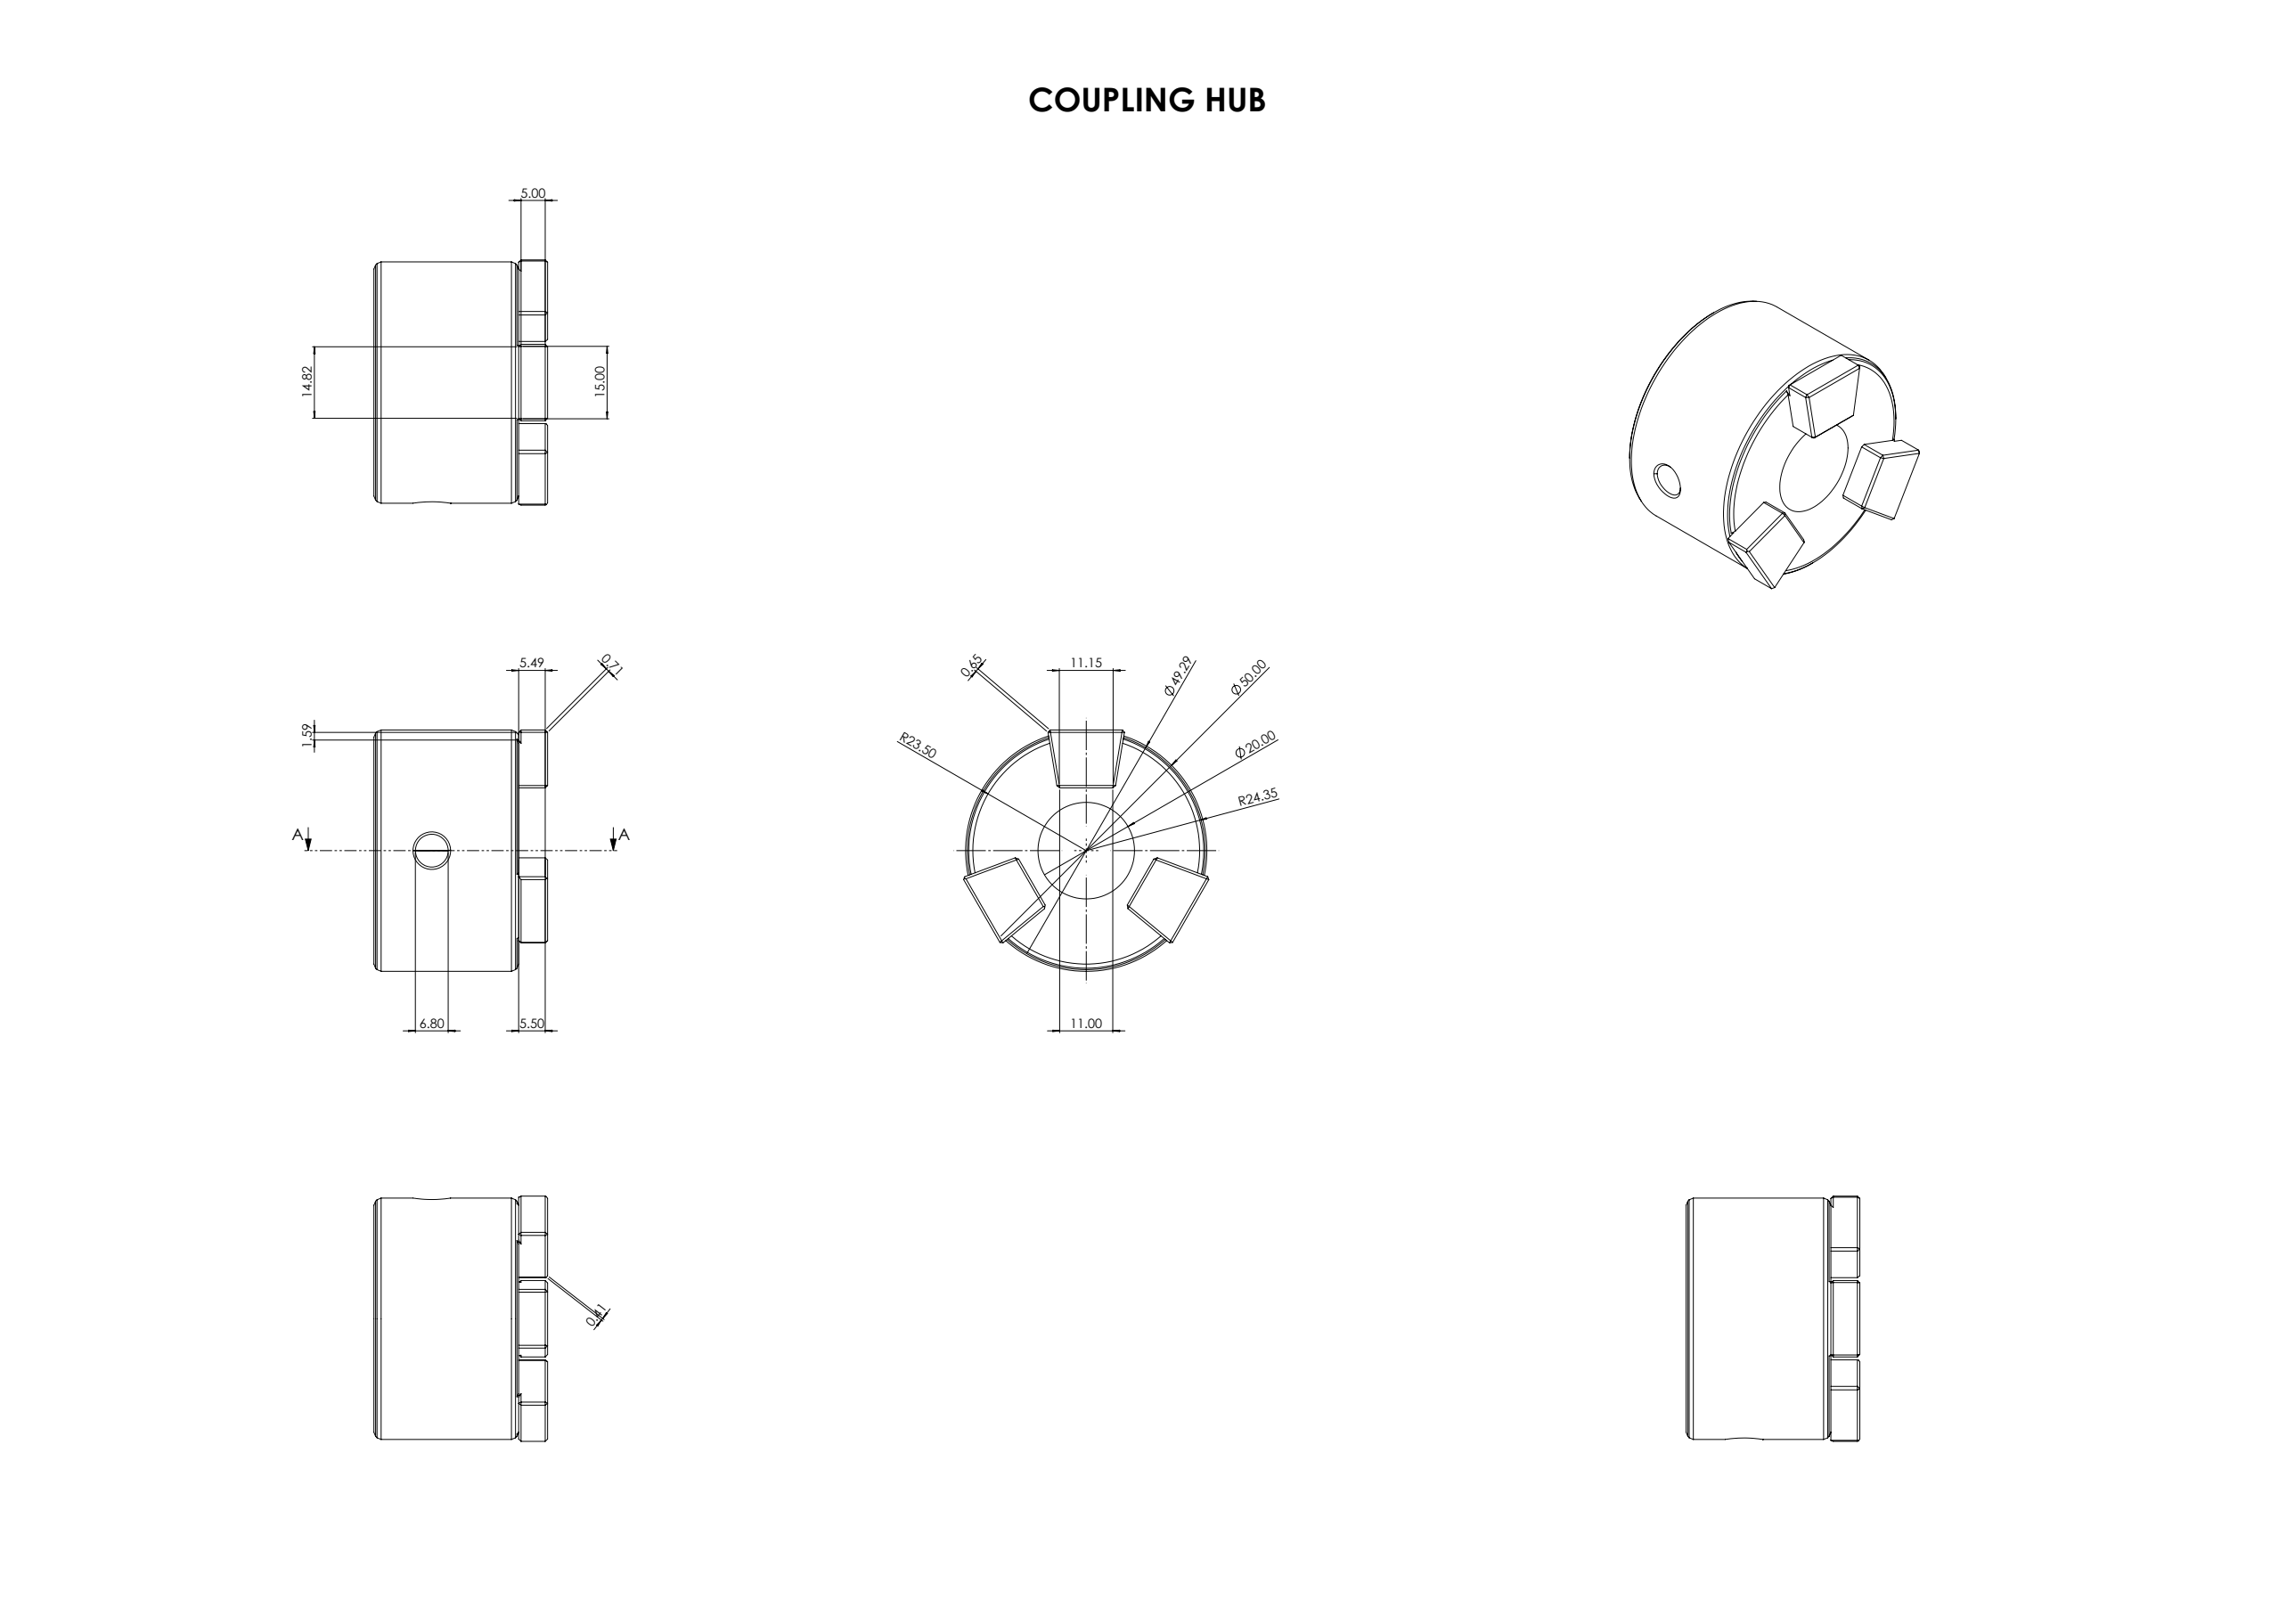
ISO-10303-21;
HEADER;
/* Generated by software containing ST-Developer
 * from STEP Tools, Inc. (www.steptools.com) 
 */

FILE_DESCRIPTION(
/* description */ (''),
/* implementation_level */ '2;1');

FILE_NAME(
/* name */ '20_Coupling_Hub.step',
/* time_stamp */ '2026-10-26T04:15:57-07:00',
/* author */ (''),
/* organization */ (''),
/* preprocessor_version */ 'ST-DEVELOPER v20.2',
/* originating_system */ 'Autodesk Translation Framework v15.15.0.0',
/* authorisation */ '');

FILE_SCHEMA (('AUTOMOTIVE_DESIGN { 1 0 10303 214 3 1 1 }'));
ENDSEC;

DATA;
#10=MECHANICAL_DESIGN_GEOMETRIC_PRESENTATION_REPRESENTATION('',(#467),#55737);
#167=(
BOUNDED_CURVE()
B_SPLINE_CURVE(2,(#46093,#46094,#46095),.UNSPECIFIED.,.F.,.F.)
B_SPLINE_CURVE_WITH_KNOTS((3,3),(0.,0.0933927438985777),.UNSPECIFIED.)
CURVE()
GEOMETRIC_REPRESENTATION_ITEM()
RATIONAL_B_SPLINE_CURVE((1.,1.00016319148553,1.))
REPRESENTATION_ITEM('')
);
#168=(
BOUNDED_CURVE()
B_SPLINE_CURVE(2,(#46101,#46102,#46103),.UNSPECIFIED.,.F.,.F.)
B_SPLINE_CURVE_WITH_KNOTS((3,3),(0.,0.0933927438985944),.UNSPECIFIED.)
CURVE()
GEOMETRIC_REPRESENTATION_ITEM()
RATIONAL_B_SPLINE_CURVE((1.,1.00016318991919,1.))
REPRESENTATION_ITEM('')
);
#169=(
BOUNDED_CURVE()
B_SPLINE_CURVE(2,(#46107,#46108,#46109),.UNSPECIFIED.,.F.,.F.)
B_SPLINE_CURVE_WITH_KNOTS((3,3),(0.0409294620252543,0.0910167227867222),
 .UNSPECIFIED.)
CURVE()
GEOMETRIC_REPRESENTATION_ITEM()
RATIONAL_B_SPLINE_CURVE((1.00010930039025,1.0001537829794,1.0001434531036))
REPRESENTATION_ITEM('')
);
#170=(
BOUNDED_CURVE()
B_SPLINE_CURVE(2,(#46116,#46117,#46118),.UNSPECIFIED.,.F.,.F.)
B_SPLINE_CURVE_WITH_KNOTS((3,3),(0.0721379811442756,0.122225241901496),
 .UNSPECIFIED.)
CURVE()
GEOMETRIC_REPRESENTATION_ITEM()
RATIONAL_B_SPLINE_CURVE((1.00014345310532,1.00015378298122,1.00010930039153))
REPRESENTATION_ITEM('')
);
#171=(
BOUNDED_CURVE()
B_SPLINE_CURVE(2,(#46120,#46121,#46122),.UNSPECIFIED.,.F.,.F.)
B_SPLINE_CURVE_WITH_KNOTS((3,3),(0.137750552840512,0.208869663053062),
 .UNSPECIFIED.)
CURVE()
GEOMETRIC_REPRESENTATION_ITEM()
RATIONAL_B_SPLINE_CURVE((1.00067579562359,1.00074006560275,1.00069056303564))
REPRESENTATION_ITEM('')
);
#172=(
BOUNDED_CURVE()
B_SPLINE_CURVE(2,(#46124,#46125,#46126),.UNSPECIFIED.,.F.,.F.)
B_SPLINE_CURVE_WITH_KNOTS((3,3),(0.190074031647834,0.281492140864205),
 .UNSPECIFIED.)
CURVE()
GEOMETRIC_REPRESENTATION_ITEM()
RATIONAL_B_SPLINE_CURVE((1.,1.,1.))
REPRESENTATION_ITEM('')
);
#173=(
BOUNDED_CURVE()
B_SPLINE_CURVE(2,(#46130,#46131,#46132),.UNSPECIFIED.,.F.,.F.)
B_SPLINE_CURVE_WITH_KNOTS((3,3),(0.232349708196804,0.282582386132944),
 .UNSPECIFIED.)
CURVE()
GEOMETRIC_REPRESENTATION_ITEM()
RATIONAL_B_SPLINE_CURVE((1.00153573820897,1.00157480000264,1.00155897131611))
REPRESENTATION_ITEM('')
);
#174=(
BOUNDED_CURVE()
B_SPLINE_CURVE(2,(#46136,#46137,#46138),.UNSPECIFIED.,.F.,.F.)
B_SPLINE_CURVE_WITH_KNOTS((3,3),(0.0721379811237271,0.122225241884583),
 .UNSPECIFIED.)
CURVE()
GEOMETRIC_REPRESENTATION_ITEM()
RATIONAL_B_SPLINE_CURVE((1.00014345306605,1.00015378293915,1.00010930036165))
REPRESENTATION_ITEM('')
);
#175=(
BOUNDED_CURVE()
B_SPLINE_CURVE(2,(#46140,#46141,#46142),.UNSPECIFIED.,.F.,.F.)
B_SPLINE_CURVE_WITH_KNOTS((3,3),(0.137750552841826,0.208869663054022),
 .UNSPECIFIED.)
CURVE()
GEOMETRIC_REPRESENTATION_ITEM()
RATIONAL_B_SPLINE_CURVE((1.00067579561801,1.00074006559664,1.00069056302993))
REPRESENTATION_ITEM('')
);
#176=(
BOUNDED_CURVE()
B_SPLINE_CURVE(2,(#46144,#46145,#46146),.UNSPECIFIED.,.F.,.F.)
B_SPLINE_CURVE_WITH_KNOTS((3,3),(0.190074031647831,0.281492140864202),
 .UNSPECIFIED.)
CURVE()
GEOMETRIC_REPRESENTATION_ITEM()
RATIONAL_B_SPLINE_CURVE((1.,1.,1.))
REPRESENTATION_ITEM('')
);
#177=(
BOUNDED_CURVE()
B_SPLINE_CURVE(2,(#46150,#46151,#46152),.UNSPECIFIED.,.F.,.F.)
B_SPLINE_CURVE_WITH_KNOTS((3,3),(0.176442821371904,0.267860930592077),
 .UNSPECIFIED.)
CURVE()
GEOMETRIC_REPRESENTATION_ITEM()
RATIONAL_B_SPLINE_CURVE((1.,1.,1.))
REPRESENTATION_ITEM('')
);
#178=(
BOUNDED_CURVE()
B_SPLINE_CURVE(2,(#46154,#46155,#46156),.UNSPECIFIED.,.F.,.F.)
B_SPLINE_CURVE_WITH_KNOTS((3,3),(0.146981648032891,0.218100758246257),
 .UNSPECIFIED.)
CURVE()
GEOMETRIC_REPRESENTATION_ITEM()
RATIONAL_B_SPLINE_CURVE((1.00069056304666,1.00074006561458,1.00067579563438))
REPRESENTATION_ITEM('')
);
#179=(
BOUNDED_CURVE()
B_SPLINE_CURVE(2,(#46158,#46159,#46160),.UNSPECIFIED.,.F.,.F.)
B_SPLINE_CURVE_WITH_KNOTS((3,3),(0.0409294620291145,0.0910167227899698),
 .UNSPECIFIED.)
CURVE()
GEOMETRIC_REPRESENTATION_ITEM()
RATIONAL_B_SPLINE_CURVE((1.00010930036165,1.00015378293915,1.00014345306605))
REPRESENTATION_ITEM('')
);
#180=(
BOUNDED_CURVE()
B_SPLINE_CURVE(2,(#46164,#46165,#46166),.UNSPECIFIED.,.F.,.F.)
B_SPLINE_CURVE_WITH_KNOTS((3,3),(0.0721379811487405,0.122225241904615),
 .UNSPECIFIED.)
CURVE()
GEOMETRIC_REPRESENTATION_ITEM()
RATIONAL_B_SPLINE_CURVE((1.00014345309917,1.00015378297462,1.00010930038684))
REPRESENTATION_ITEM('')
);
#181=(
BOUNDED_CURVE()
B_SPLINE_CURVE(2,(#46168,#46169,#46170),.UNSPECIFIED.,.F.,.F.)
B_SPLINE_CURVE_WITH_KNOTS((3,3),(0.137750552840201,0.208869663052662),
 .UNSPECIFIED.)
CURVE()
GEOMETRIC_REPRESENTATION_ITEM()
RATIONAL_B_SPLINE_CURVE((1.00067579562257,1.00074006560165,1.0006905630346))
REPRESENTATION_ITEM('')
);
#182=(
BOUNDED_CURVE()
B_SPLINE_CURVE(2,(#46172,#46173,#46174),.UNSPECIFIED.,.F.,.F.)
B_SPLINE_CURVE_WITH_KNOTS((3,3),(0.190074031647822,0.281492140864193),
 .UNSPECIFIED.)
CURVE()
GEOMETRIC_REPRESENTATION_ITEM()
RATIONAL_B_SPLINE_CURVE((1.,1.,1.))
REPRESENTATION_ITEM('')
);
#183=(
BOUNDED_CURVE()
B_SPLINE_CURVE(2,(#46178,#46179,#46180),.UNSPECIFIED.,.F.,.F.)
B_SPLINE_CURVE_WITH_KNOTS((3,3),(0.176442821371898,0.267860930592071),
 .UNSPECIFIED.)
CURVE()
GEOMETRIC_REPRESENTATION_ITEM()
RATIONAL_B_SPLINE_CURVE((1.,1.,1.))
REPRESENTATION_ITEM('')
);
#184=(
BOUNDED_CURVE()
B_SPLINE_CURVE(2,(#46181,#46182,#46183),.UNSPECIFIED.,.F.,.F.)
B_SPLINE_CURVE_WITH_KNOTS((3,3),(0.146981648038779,0.218100758251144),
 .UNSPECIFIED.)
CURVE()
GEOMETRIC_REPRESENTATION_ITEM()
RATIONAL_B_SPLINE_CURVE((1.00069056303571,1.00074006560282,1.00067579562364))
REPRESENTATION_ITEM('')
);
#185=(
BOUNDED_CURVE()
B_SPLINE_CURVE(2,(#46203,#46204,#46205),.UNSPECIFIED.,.F.,.F.)
B_SPLINE_CURVE_WITH_KNOTS((3,3),(0.500185502314131,0.592696752727807),
 .UNSPECIFIED.)
CURVE()
GEOMETRIC_REPRESENTATION_ITEM()
RATIONAL_B_SPLINE_CURVE((1.00953952216291,1.0095311894073,1.00919344691327))
REPRESENTATION_ITEM('')
);
#186=(
BOUNDED_CURVE()
B_SPLINE_CURVE(2,(#46208,#46209,#46210),.UNSPECIFIED.,.F.,.F.)
B_SPLINE_CURVE_WITH_KNOTS((3,3),(0.,0.0933927438985674),.UNSPECIFIED.)
CURVE()
GEOMETRIC_REPRESENTATION_ITEM()
RATIONAL_B_SPLINE_CURVE((1.,1.00016319114243,1.))
REPRESENTATION_ITEM('')
);
#187=(
BOUNDED_CURVE()
B_SPLINE_CURVE(2,(#46213,#46214,#46215),.UNSPECIFIED.,.F.,.F.)
B_SPLINE_CURVE_WITH_KNOTS((3,3),(0.,0.093392743898585),.UNSPECIFIED.)
CURVE()
GEOMETRIC_REPRESENTATION_ITEM()
RATIONAL_B_SPLINE_CURVE((1.,1.0001631911814,1.))
REPRESENTATION_ITEM('')
);
#188=(
BOUNDED_CURVE()
B_SPLINE_CURVE(2,(#46217,#46218,#46219),.UNSPECIFIED.,.F.,.F.)
B_SPLINE_CURVE_WITH_KNOTS((3,3),(0.,0.093392743898585),.UNSPECIFIED.)
CURVE()
GEOMETRIC_REPRESENTATION_ITEM()
RATIONAL_B_SPLINE_CURVE((1.,1.00016319331587,1.))
REPRESENTATION_ITEM('')
);
#398=CONICAL_SURFACE('',#29391,23.9267766952966,1.17809724509616);
#399=CONICAL_SURFACE('',#29395,24.5,0.785398163397442);
#400=CONICAL_SURFACE('',#29403,23.9267766952966,1.17809724509616);
#401=CONICAL_SURFACE('',#29407,24.5,0.785398163397442);
#402=CONICAL_SURFACE('',#29412,23.9267766952966,1.17809724509616);
#403=CONICAL_SURFACE('',#29414,23.9267766952966,1.17809724509616);
#404=CONICAL_SURFACE('',#29437,24.8232233047034,0.392699081698705);
#405=CONICAL_SURFACE('',#29443,24.8232233047034,0.392699081698705);
#427=SHAPE_REPRESENTATION_RELATIONSHIP('SRR','None',#55836,#447);
#447=ADVANCED_BREP_SHAPE_REPRESENTATION('',(#487),#55732);
#467=STYLED_ITEM('',(#55984),#487);
#487=MANIFOLD_SOLID_BREP('Body1',#27236);
#577=B_SPLINE_SURFACE_WITH_KNOTS('',3,3,((#46525,#46526,#46527,#46528,#46529,
#46530,#46531,#46532,#46533,#46534,#46535,#46536,#46537,#46538,#46539,#46540,
#46541,#46542,#46543,#46544,#46545,#46546,#46547,#46548,#46549,#46550,#46551,
#46552,#46553,#46554),(#46555,#46556,#46557,#46558,#46559,#46560,#46561,
#46562,#46563,#46564,#46565,#46566,#46567,#46568,#46569,#46570,#46571,#46572,
#46573,#46574,#46575,#46576,#46577,#46578,#46579,#46580,#46581,#46582,#46583,
#46584),(#46585,#46586,#46587,#46588,#46589,#46590,#46591,#46592,#46593,
#46594,#46595,#46596,#46597,#46598,#46599,#46600,#46601,#46602,#46603,#46604,
#46605,#46606,#46607,#46608,#46609,#46610,#46611,#46612,#46613,#46614),
(#46615,#46616,#46617,#46618,#46619,#46620,#46621,#46622,#46623,#46624,
#46625,#46626,#46627,#46628,#46629,#46630,#46631,#46632,#46633,#46634,#46635,
#46636,#46637,#46638,#46639,#46640,#46641,#46642,#46643,#46644)),
 .UNSPECIFIED.,.F.,.T.,.F.,(4,4),(4,2,2,1,2,1,1,1,1,1,1,1,1,1,2,1,2,2,1,
1,1,4),(0.,1.),(1.53893133527844,1.66717486055154,1.79541838582463,1.92366341643128,
2.05190844703792,2.16412209615196,2.276335745266,2.33244256982302,2.38854939438004,
2.50076304349408,2.52881645577259,2.5568698680511,2.61297669260812,2.72519034172216,
2.94961763995024,3.01374015525356,3.07786267055688,3.20610770116353,3.30229072145174,
3.39847374173995,3.44656525188405,3.59083978231636),.UNSPECIFIED.);
#713=FACE_BOUND('',#9658,.T.);
#714=FACE_BOUND('',#9684,.T.);
#715=FACE_BOUND('',#9736,.T.);
#1474=PLANE('',#29410);
#1475=PLANE('',#29416);
#1476=PLANE('',#29417);
#1477=PLANE('',#29418);
#1478=PLANE('',#29419);
#1479=PLANE('',#29420);
#1480=PLANE('',#29421);
#1481=PLANE('',#29422);
#1482=PLANE('',#29423);
#1483=PLANE('',#29424);
#1484=PLANE('',#29425);
#1485=PLANE('',#29426);
#1486=PLANE('',#29427);
#1487=PLANE('',#29428);
#1488=PLANE('',#29429);
#1489=PLANE('',#29430);
#1490=PLANE('',#29431);
#1491=PLANE('',#29432);
#1492=PLANE('',#29433);
#1493=PLANE('',#29434);
#1494=PLANE('',#29435);
#1495=PLANE('',#29436);
#1496=PLANE('',#29444);
#1497=PLANE('',#29445);
#1498=PLANE('',#29446);
#1499=PLANE('',#29447);
#1500=PLANE('',#29448);
#1501=PLANE('',#29449);
#1502=PLANE('',#29450);
#1503=PLANE('',#29451);
#1504=PLANE('',#29452);
#1505=PLANE('',#29453);
#1506=PLANE('',#29454);
#1507=PLANE('',#29455);
#1508=PLANE('',#29456);
#1509=PLANE('',#29457);
#1510=PLANE('',#29458);
#1511=PLANE('',#29459);
#1512=PLANE('',#29460);
#1513=PLANE('',#29461);
#1514=PLANE('',#29462);
#1515=PLANE('',#29463);
#1516=PLANE('',#29464);
#1517=PLANE('',#29465);
#1518=PLANE('',#29466);
#1519=PLANE('',#29467);
#1520=PLANE('',#29468);
#1521=PLANE('',#29469);
#1522=PLANE('',#29470);
#1523=PLANE('',#29471);
#1524=PLANE('',#29472);
#1525=PLANE('',#29473);
#1526=PLANE('',#29474);
#1527=PLANE('',#29475);
#1528=PLANE('',#29476);
#1529=PLANE('',#29477);
#1530=PLANE('',#29478);
#1531=PLANE('',#29479);
#1532=PLANE('',#29480);
#1533=PLANE('',#29481);
#1534=PLANE('',#29482);
#1535=PLANE('',#29486);
#1536=PLANE('',#29487);
#1537=PLANE('',#29488);
#1538=PLANE('',#29489);
#1539=PLANE('',#29490);
#1540=PLANE('',#29491);
#1541=PLANE('',#29492);
#1542=PLANE('',#29495);
#3492=LINE('',#46111,#5863);
#3493=LINE('',#46190,#5864);
#3494=LINE('',#46197,#5865);
#3495=LINE('',#46224,#5866);
#3496=LINE('',#46226,#5867);
#3497=LINE('',#46227,#5868);
#3498=LINE('',#46231,#5869);
#3499=LINE('',#46232,#5870);
#3500=LINE('',#46233,#5871);
#3501=LINE('',#46237,#5872);
#3502=LINE('',#46239,#5873);
#3503=LINE('',#46240,#5874);
#3504=LINE('',#46244,#5875);
#3505=LINE('',#46246,#5876);
#3506=LINE('',#46247,#5877);
#3507=LINE('',#46251,#5878);
#3508=LINE('',#46252,#5879);
#3509=LINE('',#46253,#5880);
#3510=LINE('',#46255,#5881);
#3511=LINE('',#46256,#5882);
#3512=LINE('',#46260,#5883);
#3513=LINE('',#46262,#5884);
#3514=LINE('',#46263,#5885);
#3515=LINE('',#46265,#5886);
#3516=LINE('',#46266,#5887);
#3517=LINE('',#46270,#5888);
#3518=LINE('',#46272,#5889);
#3519=LINE('',#46273,#5890);
#3520=LINE('',#46277,#5891);
#3521=LINE('',#46279,#5892);
#3522=LINE('',#46280,#5893);
#3523=LINE('',#46282,#5894);
#3524=LINE('',#46283,#5895);
#3525=LINE('',#46285,#5896);
#3526=LINE('',#46286,#5897);
#3527=LINE('',#46288,#5898);
#3528=LINE('',#46289,#5899);
#3529=LINE('',#46291,#5900);
#3530=LINE('',#46292,#5901);
#3531=LINE('',#46294,#5902);
#3532=LINE('',#46295,#5903);
#3533=LINE('',#46297,#5904);
#3534=LINE('',#46298,#5905);
#3535=LINE('',#46300,#5906);
#3536=LINE('',#46301,#5907);
#3537=LINE('',#46303,#5908);
#3538=LINE('',#46305,#5909);
#3539=LINE('',#46313,#5910);
#3540=LINE('',#46319,#5911);
#3541=LINE('',#46352,#5912);
#3542=LINE('',#46356,#5913);
#3543=LINE('',#46358,#5914);
#3544=LINE('',#46359,#5915);
#3545=LINE('',#46363,#5916);
#3546=LINE('',#46364,#5917);
#3547=LINE('',#46365,#5918);
#3548=LINE('',#46369,#5919);
#3549=LINE('',#46370,#5920);
#3550=LINE('',#46372,#5921);
#3551=LINE('',#46373,#5922);
#3552=LINE('',#46377,#5923);
#3553=LINE('',#46378,#5924);
#3554=LINE('',#46380,#5925);
#3555=LINE('',#46381,#5926);
#3556=LINE('',#46383,#5927);
#3557=LINE('',#46385,#5928);
#3558=LINE('',#46387,#5929);
#3559=LINE('',#46388,#5930);
#3560=LINE('',#46391,#5931);
#3561=LINE('',#46392,#5932);
#3562=LINE('',#46395,#5933);
#3563=LINE('',#46397,#5934);
#3564=LINE('',#46398,#5935);
#3565=LINE('',#46402,#5936);
#3566=LINE('',#46404,#5937);
#3567=LINE('',#46405,#5938);
#3568=LINE('',#46409,#5939);
#3569=LINE('',#46411,#5940);
#3570=LINE('',#46412,#5941);
#3571=LINE('',#46414,#5942);
#3572=LINE('',#46416,#5943);
#3573=LINE('',#46417,#5944);
#3574=LINE('',#46419,#5945);
#3575=LINE('',#46420,#5946);
#3576=LINE('',#46422,#5947);
#3577=LINE('',#46423,#5948);
#3578=LINE('',#46425,#5949);
#3579=LINE('',#46426,#5950);
#3580=LINE('',#46429,#5951);
#3581=LINE('',#46430,#5952);
#3582=LINE('',#46431,#5953);
#3583=LINE('',#46433,#5954);
#3584=LINE('',#46435,#5955);
#3585=LINE('',#46441,#5956);
#3586=LINE('',#46443,#5957);
#3587=LINE('',#46444,#5958);
#3588=LINE('',#46448,#5959);
#3589=LINE('',#46449,#5960);
#3590=LINE('',#46450,#5961);
#3591=LINE('',#46454,#5962);
#3592=LINE('',#46456,#5963);
#3593=LINE('',#46457,#5964);
#3594=LINE('',#46461,#5965);
#3595=LINE('',#46463,#5966);
#3596=LINE('',#46464,#5967);
#3597=LINE('',#46468,#5968);
#3598=LINE('',#46469,#5969);
#3599=LINE('',#46470,#5970);
#3600=LINE('',#46472,#5971);
#3601=LINE('',#46473,#5972);
#3602=LINE('',#46477,#5973);
#3603=LINE('',#46479,#5974);
#3604=LINE('',#46480,#5975);
#3605=LINE('',#46482,#5976);
#3606=LINE('',#46483,#5977);
#3607=LINE('',#46487,#5978);
#3608=LINE('',#46489,#5979);
#3609=LINE('',#46490,#5980);
#3610=LINE('',#46494,#5981);
#3611=LINE('',#46496,#5982);
#3612=LINE('',#46497,#5983);
#3613=LINE('',#46499,#5984);
#3614=LINE('',#46500,#5985);
#3615=LINE('',#46502,#5986);
#3616=LINE('',#46503,#5987);
#3617=LINE('',#46505,#5988);
#3618=LINE('',#46506,#5989);
#3619=LINE('',#46508,#5990);
#3620=LINE('',#46509,#5991);
#3621=LINE('',#46511,#5992);
#3622=LINE('',#46512,#5993);
#3623=LINE('',#46514,#5994);
#3624=LINE('',#46515,#5995);
#3625=LINE('',#46517,#5996);
#3626=LINE('',#46518,#5997);
#3627=LINE('',#46520,#5998);
#3628=LINE('',#46522,#5999);
#3629=LINE('',#46646,#6000);
#3630=LINE('',#46679,#6001);
#3631=LINE('',#46684,#6002);
#3632=LINE('',#46686,#6003);
#3633=LINE('',#46688,#6004);
#3634=LINE('',#46692,#6005);
#3635=LINE('',#46697,#6006);
#3636=LINE('',#46698,#6007);
#5863=VECTOR('',#35578,24.5);
#5864=VECTOR('',#35599,23.9267766952966);
#5865=VECTOR('',#35608,24.5);
#5866=VECTOR('',#35623,10.);
#5867=VECTOR('',#35624,10.);
#5868=VECTOR('',#35625,10.);
#5869=VECTOR('',#35628,10.);
#5870=VECTOR('',#35629,10.);
#5871=VECTOR('',#35630,10.);
#5872=VECTOR('',#35633,10.);
#5873=VECTOR('',#35634,10.);
#5874=VECTOR('',#35635,10.);
#5875=VECTOR('',#35638,10.);
#5876=VECTOR('',#35639,10.);
#5877=VECTOR('',#35640,10.);
#5878=VECTOR('',#35643,10.);
#5879=VECTOR('',#35644,10.);
#5880=VECTOR('',#35645,10.);
#5881=VECTOR('',#35648,10.);
#5882=VECTOR('',#35649,10.);
#5883=VECTOR('',#35652,10.);
#5884=VECTOR('',#35653,10.);
#5885=VECTOR('',#35654,10.);
#5886=VECTOR('',#35657,10.);
#5887=VECTOR('',#35658,10.);
#5888=VECTOR('',#35661,10.);
#5889=VECTOR('',#35662,10.);
#5890=VECTOR('',#35663,10.);
#5891=VECTOR('',#35666,10.);
#5892=VECTOR('',#35667,10.);
#5893=VECTOR('',#35668,10.);
#5894=VECTOR('',#35671,10.);
#5895=VECTOR('',#35672,10.);
#5896=VECTOR('',#35675,10.);
#5897=VECTOR('',#35676,10.);
#5898=VECTOR('',#35679,10.);
#5899=VECTOR('',#35680,10.);
#5900=VECTOR('',#35683,10.);
#5901=VECTOR('',#35684,10.);
#5902=VECTOR('',#35687,10.);
#5903=VECTOR('',#35688,10.);
#5904=VECTOR('',#35691,10.);
#5905=VECTOR('',#35692,10.);
#5906=VECTOR('',#35695,10.);
#5907=VECTOR('',#35696,10.);
#5908=VECTOR('',#35699,10.);
#5909=VECTOR('',#35702,10.);
#5910=VECTOR('',#35713,24.8232233047034);
#5911=VECTOR('',#35720,25.);
#5912=VECTOR('',#35723,24.8232233047034);
#5913=VECTOR('',#35726,10.);
#5914=VECTOR('',#35727,10.);
#5915=VECTOR('',#35728,10.);
#5916=VECTOR('',#35731,10.);
#5917=VECTOR('',#35732,10.);
#5918=VECTOR('',#35733,10.);
#5919=VECTOR('',#35736,10.);
#5920=VECTOR('',#35737,10.);
#5921=VECTOR('',#35738,10.);
#5922=VECTOR('',#35739,10.);
#5923=VECTOR('',#35742,10.);
#5924=VECTOR('',#35743,10.);
#5925=VECTOR('',#35744,10.);
#5926=VECTOR('',#35745,10.);
#5927=VECTOR('',#35748,10.);
#5928=VECTOR('',#35749,10.);
#5929=VECTOR('',#35750,10.);
#5930=VECTOR('',#35751,10.);
#5931=VECTOR('',#35754,10.);
#5932=VECTOR('',#35755,10.);
#5933=VECTOR('',#35758,10.);
#5934=VECTOR('',#35759,10.);
#5935=VECTOR('',#35760,10.);
#5936=VECTOR('',#35763,10.);
#5937=VECTOR('',#35764,10.);
#5938=VECTOR('',#35765,10.);
#5939=VECTOR('',#35768,10.);
#5940=VECTOR('',#35769,10.);
#5941=VECTOR('',#35770,10.);
#5942=VECTOR('',#35773,10.);
#5943=VECTOR('',#35774,10.);
#5944=VECTOR('',#35775,10.);
#5945=VECTOR('',#35778,10.);
#5946=VECTOR('',#35779,10.);
#5947=VECTOR('',#35782,10.);
#5948=VECTOR('',#35783,10.);
#5949=VECTOR('',#35786,10.);
#5950=VECTOR('',#35787,10.);
#5951=VECTOR('',#35790,10.);
#5952=VECTOR('',#35791,10.);
#5953=VECTOR('',#35792,10.);
#5954=VECTOR('',#35795,10.);
#5955=VECTOR('',#35798,10.);
#5956=VECTOR('',#35805,10.);
#5957=VECTOR('',#35806,10.);
#5958=VECTOR('',#35807,10.);
#5959=VECTOR('',#35810,10.);
#5960=VECTOR('',#35811,10.);
#5961=VECTOR('',#35812,10.);
#5962=VECTOR('',#35815,10.);
#5963=VECTOR('',#35816,10.);
#5964=VECTOR('',#35817,10.);
#5965=VECTOR('',#35820,10.);
#5966=VECTOR('',#35821,10.);
#5967=VECTOR('',#35822,10.);
#5968=VECTOR('',#35825,10.);
#5969=VECTOR('',#35826,10.);
#5970=VECTOR('',#35827,10.);
#5971=VECTOR('',#35830,10.);
#5972=VECTOR('',#35831,10.);
#5973=VECTOR('',#35834,10.);
#5974=VECTOR('',#35835,10.);
#5975=VECTOR('',#35836,10.);
#5976=VECTOR('',#35839,10.);
#5977=VECTOR('',#35840,10.);
#5978=VECTOR('',#35843,10.);
#5979=VECTOR('',#35844,10.);
#5980=VECTOR('',#35845,10.);
#5981=VECTOR('',#35848,10.);
#5982=VECTOR('',#35849,10.);
#5983=VECTOR('',#35850,10.);
#5984=VECTOR('',#35853,10.);
#5985=VECTOR('',#35854,10.);
#5986=VECTOR('',#35857,10.);
#5987=VECTOR('',#35858,10.);
#5988=VECTOR('',#35861,10.);
#5989=VECTOR('',#35862,10.);
#5990=VECTOR('',#35865,10.);
#5991=VECTOR('',#35866,10.);
#5992=VECTOR('',#35869,10.);
#5993=VECTOR('',#35870,10.);
#5994=VECTOR('',#35873,10.);
#5995=VECTOR('',#35874,10.);
#5996=VECTOR('',#35877,10.);
#5997=VECTOR('',#35878,10.);
#5998=VECTOR('',#35881,10.);
#5999=VECTOR('',#35884,10.);
#6000=VECTOR('',#35889,10.);
#6001=VECTOR('',#35892,3.4);
#6002=VECTOR('',#35899,10.);
#6003=VECTOR('',#35902,10.);
#6004=VECTOR('',#35905,10.);
#6005=VECTOR('',#35912,10.);
#6006=VECTOR('',#35919,10.);
#6007=VECTOR('',#35920,10.);
#6711=CYLINDRICAL_SURFACE('',#29440,25.);
#6712=CYLINDRICAL_SURFACE('',#29483,3.4);
#6713=CYLINDRICAL_SURFACE('',#29493,10.);
#7975=FACE_OUTER_BOUND('',#9653,.T.);
#7976=FACE_OUTER_BOUND('',#9654,.T.);
#7977=FACE_OUTER_BOUND('',#9655,.T.);
#7978=FACE_OUTER_BOUND('',#9656,.T.);
#7979=FACE_OUTER_BOUND('',#9657,.T.);
#7980=FACE_OUTER_BOUND('',#9659,.T.);
#7981=FACE_OUTER_BOUND('',#9660,.T.);
#7982=FACE_OUTER_BOUND('',#9661,.T.);
#7983=FACE_OUTER_BOUND('',#9662,.T.);
#7984=FACE_OUTER_BOUND('',#9663,.T.);
#7985=FACE_OUTER_BOUND('',#9664,.T.);
#7986=FACE_OUTER_BOUND('',#9665,.T.);
#7987=FACE_OUTER_BOUND('',#9666,.T.);
#7988=FACE_OUTER_BOUND('',#9667,.T.);
#7989=FACE_OUTER_BOUND('',#9668,.T.);
#7990=FACE_OUTER_BOUND('',#9669,.T.);
#7991=FACE_OUTER_BOUND('',#9670,.T.);
#7992=FACE_OUTER_BOUND('',#9671,.T.);
#7993=FACE_OUTER_BOUND('',#9672,.T.);
#7994=FACE_OUTER_BOUND('',#9673,.T.);
#7995=FACE_OUTER_BOUND('',#9674,.T.);
#7996=FACE_OUTER_BOUND('',#9675,.T.);
#7997=FACE_OUTER_BOUND('',#9676,.T.);
#7998=FACE_OUTER_BOUND('',#9677,.T.);
#7999=FACE_OUTER_BOUND('',#9678,.T.);
#8000=FACE_OUTER_BOUND('',#9679,.T.);
#8001=FACE_OUTER_BOUND('',#9680,.T.);
#8002=FACE_OUTER_BOUND('',#9681,.T.);
#8003=FACE_OUTER_BOUND('',#9682,.T.);
#8004=FACE_OUTER_BOUND('',#9683,.T.);
#8005=FACE_OUTER_BOUND('',#9685,.T.);
#8006=FACE_OUTER_BOUND('',#9686,.T.);
#8007=FACE_OUTER_BOUND('',#9687,.T.);
#8008=FACE_OUTER_BOUND('',#9688,.T.);
#8009=FACE_OUTER_BOUND('',#9689,.T.);
#8010=FACE_OUTER_BOUND('',#9690,.T.);
#8011=FACE_OUTER_BOUND('',#9691,.T.);
#8012=FACE_OUTER_BOUND('',#9692,.T.);
#8013=FACE_OUTER_BOUND('',#9693,.T.);
#8014=FACE_OUTER_BOUND('',#9694,.T.);
#8015=FACE_OUTER_BOUND('',#9695,.T.);
#8016=FACE_OUTER_BOUND('',#9696,.T.);
#8017=FACE_OUTER_BOUND('',#9697,.T.);
#8018=FACE_OUTER_BOUND('',#9698,.T.);
#8019=FACE_OUTER_BOUND('',#9699,.T.);
#8020=FACE_OUTER_BOUND('',#9700,.T.);
#8021=FACE_OUTER_BOUND('',#9701,.T.);
#8022=FACE_OUTER_BOUND('',#9702,.T.);
#8023=FACE_OUTER_BOUND('',#9703,.T.);
#8024=FACE_OUTER_BOUND('',#9704,.T.);
#8025=FACE_OUTER_BOUND('',#9705,.T.);
#8026=FACE_OUTER_BOUND('',#9706,.T.);
#8027=FACE_OUTER_BOUND('',#9707,.T.);
#8028=FACE_OUTER_BOUND('',#9708,.T.);
#8029=FACE_OUTER_BOUND('',#9709,.T.);
#8030=FACE_OUTER_BOUND('',#9710,.T.);
#8031=FACE_OUTER_BOUND('',#9711,.T.);
#8032=FACE_OUTER_BOUND('',#9712,.T.);
#8033=FACE_OUTER_BOUND('',#9713,.T.);
#8034=FACE_OUTER_BOUND('',#9714,.T.);
#8035=FACE_OUTER_BOUND('',#9715,.T.);
#8036=FACE_OUTER_BOUND('',#9716,.T.);
#8037=FACE_OUTER_BOUND('',#9717,.T.);
#8038=FACE_OUTER_BOUND('',#9718,.T.);
#8039=FACE_OUTER_BOUND('',#9719,.T.);
#8040=FACE_OUTER_BOUND('',#9720,.T.);
#8041=FACE_OUTER_BOUND('',#9721,.T.);
#8042=FACE_OUTER_BOUND('',#9722,.T.);
#8043=FACE_OUTER_BOUND('',#9723,.T.);
#8044=FACE_OUTER_BOUND('',#9724,.T.);
#8045=FACE_OUTER_BOUND('',#9725,.T.);
#8046=FACE_OUTER_BOUND('',#9726,.T.);
#8047=FACE_OUTER_BOUND('',#9727,.T.);
#8048=FACE_OUTER_BOUND('',#9728,.T.);
#8049=FACE_OUTER_BOUND('',#9729,.T.);
#8050=FACE_OUTER_BOUND('',#9730,.T.);
#8051=FACE_OUTER_BOUND('',#9731,.T.);
#8052=FACE_OUTER_BOUND('',#9732,.T.);
#8053=FACE_OUTER_BOUND('',#9733,.T.);
#8054=FACE_OUTER_BOUND('',#9734,.T.);
#8055=FACE_OUTER_BOUND('',#9735,.T.);
#9653=EDGE_LOOP('',(#23522,#23523,#23524,#23525,#23526));
#9654=EDGE_LOOP('',(#23527,#23528,#23529,#23530,#23531,#23532,#23533,#23534,
#23535,#23536,#23537,#23538,#23539,#23540,#23541,#23542,#23543,#23544,#23545,
#23546,#23547,#23548,#23549,#23550,#23551,#23552,#23553));
#9655=EDGE_LOOP('',(#23554,#23555,#23556,#23557,#23558));
#9656=EDGE_LOOP('',(#23559,#23560,#23561,#23562,#23563,#23564));
#9657=EDGE_LOOP('',(#23565));
#9658=EDGE_LOOP('',(#23566));
#9659=EDGE_LOOP('',(#23567,#23568,#23569,#23570));
#9660=EDGE_LOOP('',(#23571,#23572,#23573,#23574));
#9661=EDGE_LOOP('',(#23575,#23576,#23577));
#9662=EDGE_LOOP('',(#23578,#23579,#23580,#23581));
#9663=EDGE_LOOP('',(#23582,#23583,#23584));
#9664=EDGE_LOOP('',(#23585,#23586,#23587));
#9665=EDGE_LOOP('',(#23588,#23589,#23590,#23591));
#9666=EDGE_LOOP('',(#23592,#23593,#23594,#23595));
#9667=EDGE_LOOP('',(#23596,#23597,#23598));
#9668=EDGE_LOOP('',(#23599,#23600,#23601,#23602));
#9669=EDGE_LOOP('',(#23603,#23604,#23605));
#9670=EDGE_LOOP('',(#23606,#23607,#23608));
#9671=EDGE_LOOP('',(#23609,#23610,#23611,#23612));
#9672=EDGE_LOOP('',(#23613,#23614,#23615,#23616));
#9673=EDGE_LOOP('',(#23617,#23618,#23619,#23620));
#9674=EDGE_LOOP('',(#23621,#23622,#23623,#23624));
#9675=EDGE_LOOP('',(#23625,#23626,#23627,#23628));
#9676=EDGE_LOOP('',(#23629,#23630,#23631,#23632));
#9677=EDGE_LOOP('',(#23633,#23634,#23635,#23636));
#9678=EDGE_LOOP('',(#23637,#23638,#23639,#23640,#23641,#23642,#23643,#23644));
#9679=EDGE_LOOP('',(#23645,#23646,#23647,#23648));
#9680=EDGE_LOOP('',(#23649,#23650,#23651,#23652));
#9681=EDGE_LOOP('',(#23653,#23654,#23655,#23656));
#9682=EDGE_LOOP('',(#23657,#23658,#23659,#23660,#23661,#23662));
#9683=EDGE_LOOP('',(#23663,#23664,#23665,#23666,#23667,#23668));
#9684=EDGE_LOOP('',(#23669));
#9685=EDGE_LOOP('',(#23670,#23671,#23672,#23673,#23674,#23675));
#9686=EDGE_LOOP('',(#23676,#23677,#23678));
#9687=EDGE_LOOP('',(#23679,#23680,#23681,#23682));
#9688=EDGE_LOOP('',(#23683,#23684,#23685,#23686,#23687));
#9689=EDGE_LOOP('',(#23688,#23689,#23690,#23691,#23692));
#9690=EDGE_LOOP('',(#23693,#23694,#23695,#23696,#23697,#23698,#23699,#23700));
#9691=EDGE_LOOP('',(#23701,#23702,#23703,#23704));
#9692=EDGE_LOOP('',(#23705,#23706,#23707,#23708,#23709));
#9693=EDGE_LOOP('',(#23710,#23711,#23712));
#9694=EDGE_LOOP('',(#23713,#23714,#23715));
#9695=EDGE_LOOP('',(#23716,#23717,#23718,#23719,#23720));
#9696=EDGE_LOOP('',(#23721,#23722,#23723,#23724));
#9697=EDGE_LOOP('',(#23725,#23726,#23727,#23728));
#9698=EDGE_LOOP('',(#23729,#23730,#23731,#23732,#23733));
#9699=EDGE_LOOP('',(#23734,#23735,#23736,#23737,#23738));
#9700=EDGE_LOOP('',(#23739,#23740,#23741,#23742,#23743));
#9701=EDGE_LOOP('',(#23744,#23745,#23746,#23747,#23748,#23749,#23750,#23751));
#9702=EDGE_LOOP('',(#23752,#23753,#23754,#23755));
#9703=EDGE_LOOP('',(#23756,#23757,#23758,#23759));
#9704=EDGE_LOOP('',(#23760,#23761,#23762));
#9705=EDGE_LOOP('',(#23763,#23764,#23765,#23766));
#9706=EDGE_LOOP('',(#23767,#23768,#23769));
#9707=EDGE_LOOP('',(#23770,#23771,#23772));
#9708=EDGE_LOOP('',(#23773,#23774,#23775,#23776));
#9709=EDGE_LOOP('',(#23777,#23778,#23779,#23780));
#9710=EDGE_LOOP('',(#23781,#23782,#23783));
#9711=EDGE_LOOP('',(#23784,#23785,#23786,#23787));
#9712=EDGE_LOOP('',(#23788,#23789,#23790));
#9713=EDGE_LOOP('',(#23791,#23792,#23793));
#9714=EDGE_LOOP('',(#23794,#23795,#23796,#23797));
#9715=EDGE_LOOP('',(#23798,#23799,#23800,#23801));
#9716=EDGE_LOOP('',(#23802,#23803,#23804,#23805));
#9717=EDGE_LOOP('',(#23806,#23807,#23808,#23809));
#9718=EDGE_LOOP('',(#23810,#23811,#23812,#23813));
#9719=EDGE_LOOP('',(#23814,#23815,#23816,#23817));
#9720=EDGE_LOOP('',(#23818,#23819,#23820,#23821));
#9721=EDGE_LOOP('',(#23822,#23823,#23824,#23825,#23826,#23827,#23828,#23829));
#9722=EDGE_LOOP('',(#23830,#23831,#23832,#23833));
#9723=EDGE_LOOP('',(#23834,#23835,#23836,#23837));
#9724=EDGE_LOOP('',(#23838,#23839,#23840,#23841));
#9725=EDGE_LOOP('',(#23842,#23843,#23844,#23845));
#9726=EDGE_LOOP('',(#23846,#23847,#23848,#23849,#23850));
#9727=EDGE_LOOP('',(#23851,#23852));
#9728=EDGE_LOOP('',(#23853,#23854));
#9729=EDGE_LOOP('',(#23855,#23856,#23857,#23858,#23859,#23860,#23861,#23862));
#9730=EDGE_LOOP('',(#23863,#23864,#23865,#23866));
#9731=EDGE_LOOP('',(#23867,#23868,#23869,#23870));
#9732=EDGE_LOOP('',(#23871,#23872,#23873,#23874,#23875,#23876,#23877,#23878));
#9733=EDGE_LOOP('',(#23879,#23880,#23881,#23882));
#9734=EDGE_LOOP('',(#23883,#23884,#23885,#23886,#23887,#23888,#23889,#23890));
#9735=EDGE_LOOP('',(#23891,#23892,#23893,#23894,#23895,#23896,#23897,#23898,
#23899,#23900,#23901,#23902,#23903,#23904,#23905,#23906,#23907,#23908));
#9736=EDGE_LOOP('',(#23909));
#10847=CIRCLE('',#29392,24.3535533905933);
#10848=CIRCLE('',#29393,24.3535533905933);
#10849=CIRCLE('',#29394,23.5);
#10850=CIRCLE('',#29396,24.6464466094067);
#10851=CIRCLE('',#29397,24.6464466094067);
#10852=CIRCLE('',#29398,24.);
#10853=CIRCLE('',#29399,24.3535533905933);
#10854=CIRCLE('',#29400,24.);
#10855=CIRCLE('',#29401,24.3535533905933);
#10856=CIRCLE('',#29402,24.);
#10857=CIRCLE('',#29404,24.3535533905933);
#10858=CIRCLE('',#29405,24.3535533905933);
#10859=CIRCLE('',#29406,23.5);
#10860=CIRCLE('',#29408,24.6464466094067);
#10861=CIRCLE('',#29409,24.6464466094067);
#10862=CIRCLE('',#29411,10.);
#10863=CIRCLE('',#29413,23.5);
#10864=CIRCLE('',#29415,23.5);
#10865=CIRCLE('',#29438,25.);
#10866=CIRCLE('',#29439,25.);
#10867=CIRCLE('',#29441,25.);
#10868=CIRCLE('',#29442,25.);
#10869=CIRCLE('',#29484,3.4);
#10870=CIRCLE('',#29485,3.4);
#10871=CIRCLE('',#29494,10.);
#11223=B_SPLINE_CURVE_WITH_KNOTS('',3,(#46321,#46322,#46323,#46324,#46325,
#46326,#46327,#46328,#46329,#46330,#46331,#46332,#46333,#46334,#46335,#46336,
#46337,#46338,#46339,#46340,#46341,#46342,#46343,#46344,#46345,#46346,#46347,
#46348,#46349,#46350),.UNSPECIFIED.,.T.,.F.,(4,1,1,1,2,2,1,2,1,1,1,1,1,
1,1,1,1,2,1,2,2,4),(-3.59083978231636,-3.44656525188405,-3.39847374173995,
-3.30229072145174,-3.20610770116353,-3.07786267055688,-3.01374015525356,
-2.94961763995024,-2.72519034172216,-2.61297669260812,-2.5568698680511,
-2.52881645577259,-2.50076304349408,-2.38854939438004,-2.33244256982302,
-2.276335745266,-2.16412209615196,-2.05190844703792,-1.92366341643128,-1.79541838582463,
-1.66717486055154,-1.53893133527844),.UNSPECIFIED.);
#11224=B_SPLINE_CURVE_WITH_KNOTS('',3,(#46647,#46648,#46649,#46650,#46651,
#46652,#46653,#46654,#46655,#46656,#46657,#46658,#46659,#46660,#46661,#46662,
#46663,#46664,#46665,#46666,#46667,#46668,#46669,#46670,#46671,#46672,#46673,
#46674,#46675,#46676),.UNSPECIFIED.,.T.,.F.,(4,2,2,1,2,1,1,1,1,1,1,1,1,
1,2,1,2,2,1,1,1,4),(1.53893133527844,1.66717486055154,1.79541838582463,
1.92366341643128,2.05190844703792,2.16412209615196,2.276335745266,2.33244256982302,
2.38854939438004,2.50076304349408,2.52881645577259,2.5568698680511,2.61297669260812,
2.72519034172216,2.94961763995024,3.01374015525356,3.07786267055688,3.20610770116353,
3.30229072145174,3.39847374173995,3.44656525188405,3.59083978231636),
 .UNSPECIFIED.);
#13240=VERTEX_POINT('',#46091);
#13241=VERTEX_POINT('',#46092);
#13242=VERTEX_POINT('',#46096);
#13243=VERTEX_POINT('',#46098);
#13244=VERTEX_POINT('',#46100);
#13245=VERTEX_POINT('',#46106);
#13246=VERTEX_POINT('',#46110);
#13247=VERTEX_POINT('',#46112);
#13248=VERTEX_POINT('',#46115);
#13249=VERTEX_POINT('',#46119);
#13250=VERTEX_POINT('',#46123);
#13251=VERTEX_POINT('',#46127);
#13252=VERTEX_POINT('',#46129);
#13253=VERTEX_POINT('',#46133);
#13254=VERTEX_POINT('',#46135);
#13255=VERTEX_POINT('',#46139);
#13256=VERTEX_POINT('',#46143);
#13257=VERTEX_POINT('',#46147);
#13258=VERTEX_POINT('',#46149);
#13259=VERTEX_POINT('',#46153);
#13260=VERTEX_POINT('',#46157);
#13261=VERTEX_POINT('',#46161);
#13262=VERTEX_POINT('',#46163);
#13263=VERTEX_POINT('',#46167);
#13264=VERTEX_POINT('',#46171);
#13265=VERTEX_POINT('',#46175);
#13266=VERTEX_POINT('',#46177);
#13267=VERTEX_POINT('',#46185);
#13268=VERTEX_POINT('',#46186);
#13269=VERTEX_POINT('',#46189);
#13270=VERTEX_POINT('',#46193);
#13271=VERTEX_POINT('',#46194);
#13272=VERTEX_POINT('',#46199);
#13273=VERTEX_POINT('',#46202);
#13274=VERTEX_POINT('',#46206);
#13275=VERTEX_POINT('',#46212);
#13276=VERTEX_POINT('',#46216);
#13277=VERTEX_POINT('',#46222);
#13278=VERTEX_POINT('',#46223);
#13279=VERTEX_POINT('',#46225);
#13280=VERTEX_POINT('',#46229);
#13281=VERTEX_POINT('',#46230);
#13282=VERTEX_POINT('',#46235);
#13283=VERTEX_POINT('',#46236);
#13284=VERTEX_POINT('',#46238);
#13285=VERTEX_POINT('',#46242);
#13286=VERTEX_POINT('',#46243);
#13287=VERTEX_POINT('',#46245);
#13288=VERTEX_POINT('',#46249);
#13289=VERTEX_POINT('',#46250);
#13290=VERTEX_POINT('',#46258);
#13291=VERTEX_POINT('',#46259);
#13292=VERTEX_POINT('',#46261);
#13293=VERTEX_POINT('',#46268);
#13294=VERTEX_POINT('',#46269);
#13295=VERTEX_POINT('',#46271);
#13296=VERTEX_POINT('',#46275);
#13297=VERTEX_POINT('',#46276);
#13298=VERTEX_POINT('',#46278);
#13299=VERTEX_POINT('',#46309);
#13300=VERTEX_POINT('',#46310);
#13301=VERTEX_POINT('',#46315);
#13302=VERTEX_POINT('',#46316);
#13303=VERTEX_POINT('',#46320);
#13304=VERTEX_POINT('',#46354);
#13305=VERTEX_POINT('',#46355);
#13306=VERTEX_POINT('',#46357);
#13307=VERTEX_POINT('',#46361);
#13308=VERTEX_POINT('',#46362);
#13309=VERTEX_POINT('',#46367);
#13310=VERTEX_POINT('',#46368);
#13311=VERTEX_POINT('',#46371);
#13312=VERTEX_POINT('',#46375);
#13313=VERTEX_POINT('',#46376);
#13314=VERTEX_POINT('',#46379);
#13315=VERTEX_POINT('',#46384);
#13316=VERTEX_POINT('',#46386);
#13317=VERTEX_POINT('',#46390);
#13318=VERTEX_POINT('',#46394);
#13319=VERTEX_POINT('',#46396);
#13320=VERTEX_POINT('',#46400);
#13321=VERTEX_POINT('',#46401);
#13322=VERTEX_POINT('',#46403);
#13323=VERTEX_POINT('',#46407);
#13324=VERTEX_POINT('',#46408);
#13325=VERTEX_POINT('',#46410);
#13326=VERTEX_POINT('',#46415);
#13327=VERTEX_POINT('',#46428);
#13328=VERTEX_POINT('',#46439);
#13329=VERTEX_POINT('',#46440);
#13330=VERTEX_POINT('',#46442);
#13331=VERTEX_POINT('',#46446);
#13332=VERTEX_POINT('',#46447);
#13333=VERTEX_POINT('',#46452);
#13334=VERTEX_POINT('',#46453);
#13335=VERTEX_POINT('',#46455);
#13336=VERTEX_POINT('',#46459);
#13337=VERTEX_POINT('',#46460);
#13338=VERTEX_POINT('',#46462);
#13339=VERTEX_POINT('',#46466);
#13340=VERTEX_POINT('',#46467);
#13341=VERTEX_POINT('',#46475);
#13342=VERTEX_POINT('',#46476);
#13343=VERTEX_POINT('',#46478);
#13344=VERTEX_POINT('',#46485);
#13345=VERTEX_POINT('',#46486);
#13346=VERTEX_POINT('',#46488);
#13347=VERTEX_POINT('',#46492);
#13348=VERTEX_POINT('',#46493);
#13349=VERTEX_POINT('',#46495);
#13350=VERTEX_POINT('',#46645);
#13351=VERTEX_POINT('',#46678);
#13352=VERTEX_POINT('',#46680);
#13353=VERTEX_POINT('',#46695);
#16765=EDGE_CURVE('',#13240,#13241,#167,.F.);
#16766=EDGE_CURVE('',#13241,#13242,#10847,.T.);
#16767=EDGE_CURVE('',#13242,#13243,#10848,.T.);
#16768=EDGE_CURVE('',#13243,#13244,#168,.F.);
#16769=EDGE_CURVE('',#13244,#13240,#10849,.T.);
#16770=EDGE_CURVE('',#13243,#13245,#169,.T.);
#16771=EDGE_CURVE('',#13242,#13246,#3492,.T.);
#16772=EDGE_CURVE('',#13247,#13246,#10850,.T.);
#16773=EDGE_CURVE('',#13246,#13247,#10851,.T.);
#16774=EDGE_CURVE('',#13248,#13241,#170,.T.);
#16775=EDGE_CURVE('',#13248,#13249,#171,.T.);
#16776=EDGE_CURVE('',#13249,#13250,#172,.T.);
#16777=EDGE_CURVE('',#13251,#13250,#10852,.T.);
#16778=EDGE_CURVE('',#13252,#13251,#173,.T.);
#16779=EDGE_CURVE('',#13253,#13252,#10853,.T.);
#16780=EDGE_CURVE('',#13254,#13253,#174,.T.);
#16781=EDGE_CURVE('',#13254,#13255,#175,.T.);
#16782=EDGE_CURVE('',#13255,#13256,#176,.T.);
#16783=EDGE_CURVE('',#13257,#13256,#10854,.T.);
#16784=EDGE_CURVE('',#13258,#13257,#177,.F.);
#16785=EDGE_CURVE('',#13258,#13259,#178,.T.);
#16786=EDGE_CURVE('',#13260,#13259,#179,.T.);
#16787=EDGE_CURVE('',#13261,#13260,#10855,.T.);
#16788=EDGE_CURVE('',#13262,#13261,#180,.T.);
#16789=EDGE_CURVE('',#13262,#13263,#181,.T.);
#16790=EDGE_CURVE('',#13263,#13264,#182,.T.);
#16791=EDGE_CURVE('',#13265,#13264,#10856,.T.);
#16792=EDGE_CURVE('',#13266,#13265,#183,.F.);
#16793=EDGE_CURVE('',#13266,#13245,#184,.T.);
#16794=EDGE_CURVE('',#13267,#13268,#10857,.T.);
#16795=EDGE_CURVE('',#13268,#13267,#10858,.T.);
#16796=EDGE_CURVE('',#13267,#13269,#3493,.T.);
#16797=EDGE_CURVE('',#13269,#13269,#10859,.T.);
#16798=EDGE_CURVE('',#13270,#13271,#10860,.T.);
#16799=EDGE_CURVE('',#13271,#13270,#10861,.T.);
#16800=EDGE_CURVE('',#13271,#13268,#3494,.T.);
#16801=EDGE_CURVE('',#13272,#13272,#10862,.T.);
#16802=EDGE_CURVE('',#13252,#13273,#185,.F.);
#16803=EDGE_CURVE('',#13273,#13274,#10863,.T.);
#16804=EDGE_CURVE('',#13274,#13253,#186,.F.);
#16805=EDGE_CURVE('',#13275,#13261,#187,.F.);
#16806=EDGE_CURVE('',#13260,#13276,#188,.F.);
#16807=EDGE_CURVE('',#13276,#13275,#10864,.T.);
#16808=EDGE_CURVE('',#13277,#13278,#3495,.T.);
#16809=EDGE_CURVE('',#13279,#13277,#3496,.T.);
#16810=EDGE_CURVE('',#13278,#13279,#3497,.T.);
#16811=EDGE_CURVE('',#13280,#13281,#3498,.F.);
#16812=EDGE_CURVE('',#13281,#13279,#3499,.T.);
#16813=EDGE_CURVE('',#13277,#13280,#3500,.T.);
#16814=EDGE_CURVE('',#13282,#13283,#3501,.T.);
#16815=EDGE_CURVE('',#13284,#13282,#3502,.T.);
#16816=EDGE_CURVE('',#13283,#13284,#3503,.T.);
#16817=EDGE_CURVE('',#13285,#13286,#3504,.T.);
#16818=EDGE_CURVE('',#13287,#13285,#3505,.T.);
#16819=EDGE_CURVE('',#13286,#13287,#3506,.T.);
#16820=EDGE_CURVE('',#13288,#13289,#3507,.F.);
#16821=EDGE_CURVE('',#13289,#13287,#3508,.T.);
#16822=EDGE_CURVE('',#13285,#13288,#3509,.T.);
#16823=EDGE_CURVE('',#13278,#13286,#3510,.T.);
#16824=EDGE_CURVE('',#13287,#13277,#3511,.T.);
#16825=EDGE_CURVE('',#13290,#13291,#3512,.T.);
#16826=EDGE_CURVE('',#13292,#13290,#3513,.T.);
#16827=EDGE_CURVE('',#13291,#13292,#3514,.T.);
#16828=EDGE_CURVE('',#13257,#13292,#3515,.T.);
#16829=EDGE_CURVE('',#13290,#13258,#3516,.T.);
#16830=EDGE_CURVE('',#13293,#13294,#3517,.T.);
#16831=EDGE_CURVE('',#13295,#13293,#3518,.T.);
#16832=EDGE_CURVE('',#13294,#13295,#3519,.T.);
#16833=EDGE_CURVE('',#13296,#13297,#3520,.T.);
#16834=EDGE_CURVE('',#13298,#13296,#3521,.T.);
#16835=EDGE_CURVE('',#13297,#13298,#3522,.T.);
#16836=EDGE_CURVE('',#13296,#13291,#3523,.T.);
#16837=EDGE_CURVE('',#13292,#13298,#3524,.T.);
#16838=EDGE_CURVE('',#13255,#13297,#3525,.T.);
#16839=EDGE_CURVE('',#13298,#13256,#3526,.T.);
#16840=EDGE_CURVE('',#13293,#13296,#3527,.T.);
#16841=EDGE_CURVE('',#13297,#13295,#3528,.T.);
#16842=EDGE_CURVE('',#13286,#13294,#3529,.T.);
#16843=EDGE_CURVE('',#13295,#13285,#3530,.T.);
#16844=EDGE_CURVE('',#13294,#13283,#3531,.T.);
#16845=EDGE_CURVE('',#13284,#13293,#3532,.T.);
#16846=EDGE_CURVE('',#13282,#13290,#3533,.T.);
#16847=EDGE_CURVE('',#13291,#13284,#3534,.T.);
#16848=EDGE_CURVE('',#13283,#13278,#3535,.T.);
#16849=EDGE_CURVE('',#13279,#13282,#3536,.T.);
#16850=EDGE_CURVE('',#13276,#13281,#3537,.T.);
#16851=EDGE_CURVE('',#13280,#13289,#3538,.T.);
#16852=EDGE_CURVE('',#13299,#13300,#10865,.T.);
#16853=EDGE_CURVE('',#13300,#13299,#10866,.T.);
#16854=EDGE_CURVE('',#13299,#13270,#3539,.T.);
#16855=EDGE_CURVE('',#13301,#13302,#10867,.T.);
#16856=EDGE_CURVE('',#13302,#13301,#10868,.T.);
#16857=EDGE_CURVE('',#13302,#13300,#3540,.T.);
#16858=EDGE_CURVE('',#13303,#13303,#11223,.T.);
#16859=EDGE_CURVE('',#13247,#13301,#3541,.T.);
#16860=EDGE_CURVE('',#13304,#13305,#3542,.T.);
#16861=EDGE_CURVE('',#13306,#13304,#3543,.T.);
#16862=EDGE_CURVE('',#13305,#13306,#3544,.T.);
#16863=EDGE_CURVE('',#13307,#13308,#3545,.F.);
#16864=EDGE_CURVE('',#13308,#13306,#3546,.T.);
#16865=EDGE_CURVE('',#13304,#13307,#3547,.T.);
#16866=EDGE_CURVE('',#13309,#13310,#3548,.T.);
#16867=EDGE_CURVE('',#13310,#13305,#3549,.T.);
#16868=EDGE_CURVE('',#13306,#13311,#3550,.T.);
#16869=EDGE_CURVE('',#13311,#13309,#3551,.T.);
#16870=EDGE_CURVE('',#13312,#13313,#3552,.T.);
#16871=EDGE_CURVE('',#13313,#13304,#3553,.T.);
#16872=EDGE_CURVE('',#13305,#13314,#3554,.T.);
#16873=EDGE_CURVE('',#13314,#13312,#3555,.T.);
#16874=EDGE_CURVE('',#13273,#13308,#3556,.T.);
#16875=EDGE_CURVE('',#13251,#13315,#3557,.T.);
#16876=EDGE_CURVE('',#13316,#13315,#3558,.T.);
#16877=EDGE_CURVE('',#13311,#13316,#3559,.T.);
#16878=EDGE_CURVE('',#13317,#13313,#3560,.T.);
#16879=EDGE_CURVE('',#13307,#13317,#3561,.T.);
#16880=EDGE_CURVE('',#13312,#13318,#3562,.T.);
#16881=EDGE_CURVE('',#13318,#13319,#3563,.T.);
#16882=EDGE_CURVE('',#13319,#13317,#3564,.F.);
#16883=EDGE_CURVE('',#13320,#13321,#3565,.T.);
#16884=EDGE_CURVE('',#13322,#13320,#3566,.T.);
#16885=EDGE_CURVE('',#13321,#13322,#3567,.T.);
#16886=EDGE_CURVE('',#13323,#13324,#3568,.T.);
#16887=EDGE_CURVE('',#13325,#13323,#3569,.T.);
#16888=EDGE_CURVE('',#13324,#13325,#3570,.T.);
#16889=EDGE_CURVE('',#13315,#13325,#3571,.T.);
#16890=EDGE_CURVE('',#13323,#13326,#3572,.T.);
#16891=EDGE_CURVE('',#13326,#13316,#3573,.T.);
#16892=EDGE_CURVE('',#13249,#13324,#3574,.T.);
#16893=EDGE_CURVE('',#13325,#13250,#3575,.T.);
#16894=EDGE_CURVE('',#13320,#13323,#3576,.T.);
#16895=EDGE_CURVE('',#13324,#13322,#3577,.T.);
#16896=EDGE_CURVE('',#13314,#13321,#3578,.T.);
#16897=EDGE_CURVE('',#13322,#13318,#3579,.T.);
#16898=EDGE_CURVE('',#13327,#13309,#3580,.T.);
#16899=EDGE_CURVE('',#13327,#13320,#3581,.T.);
#16900=EDGE_CURVE('',#13321,#13310,#3582,.T.);
#16901=EDGE_CURVE('',#13326,#13327,#3583,.T.);
#16902=EDGE_CURVE('',#13319,#13240,#3584,.T.);
#16903=EDGE_CURVE('',#13328,#13329,#3585,.T.);
#16904=EDGE_CURVE('',#13330,#13328,#3586,.T.);
#16905=EDGE_CURVE('',#13329,#13330,#3587,.T.);
#16906=EDGE_CURVE('',#13331,#13332,#3588,.F.);
#16907=EDGE_CURVE('',#13332,#13330,#3589,.T.);
#16908=EDGE_CURVE('',#13328,#13331,#3590,.T.);
#16909=EDGE_CURVE('',#13333,#13334,#3591,.T.);
#16910=EDGE_CURVE('',#13335,#13333,#3592,.T.);
#16911=EDGE_CURVE('',#13334,#13335,#3593,.T.);
#16912=EDGE_CURVE('',#13336,#13337,#3594,.T.);
#16913=EDGE_CURVE('',#13338,#13336,#3595,.T.);
#16914=EDGE_CURVE('',#13337,#13338,#3596,.T.);
#16915=EDGE_CURVE('',#13339,#13340,#3597,.F.);
#16916=EDGE_CURVE('',#13340,#13338,#3598,.T.);
#16917=EDGE_CURVE('',#13336,#13339,#3599,.T.);
#16918=EDGE_CURVE('',#13329,#13337,#3600,.T.);
#16919=EDGE_CURVE('',#13338,#13328,#3601,.T.);
#16920=EDGE_CURVE('',#13341,#13342,#3602,.T.);
#16921=EDGE_CURVE('',#13343,#13341,#3603,.T.);
#16922=EDGE_CURVE('',#13342,#13343,#3604,.T.);
#16923=EDGE_CURVE('',#13265,#13343,#3605,.T.);
#16924=EDGE_CURVE('',#13341,#13266,#3606,.T.);
#16925=EDGE_CURVE('',#13344,#13345,#3607,.T.);
#16926=EDGE_CURVE('',#13346,#13344,#3608,.T.);
#16927=EDGE_CURVE('',#13345,#13346,#3609,.T.);
#16928=EDGE_CURVE('',#13347,#13348,#3610,.T.);
#16929=EDGE_CURVE('',#13349,#13347,#3611,.T.);
#16930=EDGE_CURVE('',#13348,#13349,#3612,.T.);
#16931=EDGE_CURVE('',#13347,#13342,#3613,.T.);
#16932=EDGE_CURVE('',#13343,#13349,#3614,.T.);
#16933=EDGE_CURVE('',#13263,#13348,#3615,.T.);
#16934=EDGE_CURVE('',#13349,#13264,#3616,.T.);
#16935=EDGE_CURVE('',#13344,#13347,#3617,.T.);
#16936=EDGE_CURVE('',#13348,#13346,#3618,.T.);
#16937=EDGE_CURVE('',#13337,#13345,#3619,.T.);
#16938=EDGE_CURVE('',#13346,#13336,#3620,.T.);
#16939=EDGE_CURVE('',#13345,#13334,#3621,.T.);
#16940=EDGE_CURVE('',#13335,#13344,#3622,.T.);
#16941=EDGE_CURVE('',#13333,#13341,#3623,.T.);
#16942=EDGE_CURVE('',#13342,#13335,#3624,.T.);
#16943=EDGE_CURVE('',#13334,#13329,#3625,.T.);
#16944=EDGE_CURVE('',#13330,#13333,#3626,.T.);
#16945=EDGE_CURVE('',#13244,#13332,#3627,.T.);
#16946=EDGE_CURVE('',#13331,#13340,#3628,.T.);
#16947=EDGE_CURVE('',#13303,#13350,#3629,.T.);
#16948=EDGE_CURVE('',#13350,#13350,#11224,.T.);
#16949=EDGE_CURVE('',#13350,#13351,#3630,.T.);
#16950=EDGE_CURVE('',#13351,#13352,#10869,.T.);
#16951=EDGE_CURVE('',#13352,#13351,#10870,.T.);
#16952=EDGE_CURVE('',#13352,#13351,#3631,.T.);
#16953=EDGE_CURVE('',#13352,#13351,#3632,.T.);
#16954=EDGE_CURVE('',#13339,#13275,#3633,.T.);
#16955=EDGE_CURVE('',#13288,#13274,#3634,.T.);
#16956=EDGE_CURVE('',#13353,#13353,#10871,.T.);
#16957=EDGE_CURVE('',#13353,#13352,#3635,.T.);
#16958=EDGE_CURVE('',#13351,#13272,#3636,.T.);
#23522=ORIENTED_EDGE('',*,*,#16765,.T.);
#23523=ORIENTED_EDGE('',*,*,#16766,.T.);
#23524=ORIENTED_EDGE('',*,*,#16767,.T.);
#23525=ORIENTED_EDGE('',*,*,#16768,.T.);
#23526=ORIENTED_EDGE('',*,*,#16769,.T.);
#23527=ORIENTED_EDGE('',*,*,#16770,.F.);
#23528=ORIENTED_EDGE('',*,*,#16767,.F.);
#23529=ORIENTED_EDGE('',*,*,#16771,.T.);
#23530=ORIENTED_EDGE('',*,*,#16772,.F.);
#23531=ORIENTED_EDGE('',*,*,#16773,.F.);
#23532=ORIENTED_EDGE('',*,*,#16771,.F.);
#23533=ORIENTED_EDGE('',*,*,#16766,.F.);
#23534=ORIENTED_EDGE('',*,*,#16774,.F.);
#23535=ORIENTED_EDGE('',*,*,#16775,.T.);
#23536=ORIENTED_EDGE('',*,*,#16776,.T.);
#23537=ORIENTED_EDGE('',*,*,#16777,.F.);
#23538=ORIENTED_EDGE('',*,*,#16778,.F.);
#23539=ORIENTED_EDGE('',*,*,#16779,.F.);
#23540=ORIENTED_EDGE('',*,*,#16780,.F.);
#23541=ORIENTED_EDGE('',*,*,#16781,.T.);
#23542=ORIENTED_EDGE('',*,*,#16782,.T.);
#23543=ORIENTED_EDGE('',*,*,#16783,.F.);
#23544=ORIENTED_EDGE('',*,*,#16784,.F.);
#23545=ORIENTED_EDGE('',*,*,#16785,.T.);
#23546=ORIENTED_EDGE('',*,*,#16786,.F.);
#23547=ORIENTED_EDGE('',*,*,#16787,.F.);
#23548=ORIENTED_EDGE('',*,*,#16788,.F.);
#23549=ORIENTED_EDGE('',*,*,#16789,.T.);
#23550=ORIENTED_EDGE('',*,*,#16790,.T.);
#23551=ORIENTED_EDGE('',*,*,#16791,.F.);
#23552=ORIENTED_EDGE('',*,*,#16792,.F.);
#23553=ORIENTED_EDGE('',*,*,#16793,.T.);
#23554=ORIENTED_EDGE('',*,*,#16794,.T.);
#23555=ORIENTED_EDGE('',*,*,#16795,.T.);
#23556=ORIENTED_EDGE('',*,*,#16796,.T.);
#23557=ORIENTED_EDGE('',*,*,#16797,.T.);
#23558=ORIENTED_EDGE('',*,*,#16796,.F.);
#23559=ORIENTED_EDGE('',*,*,#16798,.F.);
#23560=ORIENTED_EDGE('',*,*,#16799,.F.);
#23561=ORIENTED_EDGE('',*,*,#16800,.T.);
#23562=ORIENTED_EDGE('',*,*,#16794,.F.);
#23563=ORIENTED_EDGE('',*,*,#16795,.F.);
#23564=ORIENTED_EDGE('',*,*,#16800,.F.);
#23565=ORIENTED_EDGE('',*,*,#16797,.F.);
#23566=ORIENTED_EDGE('',*,*,#16801,.T.);
#23567=ORIENTED_EDGE('',*,*,#16802,.T.);
#23568=ORIENTED_EDGE('',*,*,#16803,.T.);
#23569=ORIENTED_EDGE('',*,*,#16804,.T.);
#23570=ORIENTED_EDGE('',*,*,#16779,.T.);
#23571=ORIENTED_EDGE('',*,*,#16805,.T.);
#23572=ORIENTED_EDGE('',*,*,#16787,.T.);
#23573=ORIENTED_EDGE('',*,*,#16806,.T.);
#23574=ORIENTED_EDGE('',*,*,#16807,.T.);
#23575=ORIENTED_EDGE('',*,*,#16808,.F.);
#23576=ORIENTED_EDGE('',*,*,#16809,.F.);
#23577=ORIENTED_EDGE('',*,*,#16810,.F.);
#23578=ORIENTED_EDGE('',*,*,#16811,.T.);
#23579=ORIENTED_EDGE('',*,*,#16812,.T.);
#23580=ORIENTED_EDGE('',*,*,#16809,.T.);
#23581=ORIENTED_EDGE('',*,*,#16813,.T.);
#23582=ORIENTED_EDGE('',*,*,#16814,.F.);
#23583=ORIENTED_EDGE('',*,*,#16815,.F.);
#23584=ORIENTED_EDGE('',*,*,#16816,.F.);
#23585=ORIENTED_EDGE('',*,*,#16817,.F.);
#23586=ORIENTED_EDGE('',*,*,#16818,.F.);
#23587=ORIENTED_EDGE('',*,*,#16819,.F.);
#23588=ORIENTED_EDGE('',*,*,#16820,.T.);
#23589=ORIENTED_EDGE('',*,*,#16821,.T.);
#23590=ORIENTED_EDGE('',*,*,#16818,.T.);
#23591=ORIENTED_EDGE('',*,*,#16822,.T.);
#23592=ORIENTED_EDGE('',*,*,#16808,.T.);
#23593=ORIENTED_EDGE('',*,*,#16823,.T.);
#23594=ORIENTED_EDGE('',*,*,#16819,.T.);
#23595=ORIENTED_EDGE('',*,*,#16824,.T.);
#23596=ORIENTED_EDGE('',*,*,#16825,.F.);
#23597=ORIENTED_EDGE('',*,*,#16826,.F.);
#23598=ORIENTED_EDGE('',*,*,#16827,.F.);
#23599=ORIENTED_EDGE('',*,*,#16784,.T.);
#23600=ORIENTED_EDGE('',*,*,#16828,.T.);
#23601=ORIENTED_EDGE('',*,*,#16826,.T.);
#23602=ORIENTED_EDGE('',*,*,#16829,.T.);
#23603=ORIENTED_EDGE('',*,*,#16830,.F.);
#23604=ORIENTED_EDGE('',*,*,#16831,.F.);
#23605=ORIENTED_EDGE('',*,*,#16832,.F.);
#23606=ORIENTED_EDGE('',*,*,#16833,.F.);
#23607=ORIENTED_EDGE('',*,*,#16834,.F.);
#23608=ORIENTED_EDGE('',*,*,#16835,.F.);
#23609=ORIENTED_EDGE('',*,*,#16834,.T.);
#23610=ORIENTED_EDGE('',*,*,#16836,.T.);
#23611=ORIENTED_EDGE('',*,*,#16827,.T.);
#23612=ORIENTED_EDGE('',*,*,#16837,.T.);
#23613=ORIENTED_EDGE('',*,*,#16782,.F.);
#23614=ORIENTED_EDGE('',*,*,#16838,.T.);
#23615=ORIENTED_EDGE('',*,*,#16835,.T.);
#23616=ORIENTED_EDGE('',*,*,#16839,.T.);
#23617=ORIENTED_EDGE('',*,*,#16831,.T.);
#23618=ORIENTED_EDGE('',*,*,#16840,.T.);
#23619=ORIENTED_EDGE('',*,*,#16833,.T.);
#23620=ORIENTED_EDGE('',*,*,#16841,.T.);
#23621=ORIENTED_EDGE('',*,*,#16817,.T.);
#23622=ORIENTED_EDGE('',*,*,#16842,.T.);
#23623=ORIENTED_EDGE('',*,*,#16832,.T.);
#23624=ORIENTED_EDGE('',*,*,#16843,.T.);
#23625=ORIENTED_EDGE('',*,*,#16830,.T.);
#23626=ORIENTED_EDGE('',*,*,#16844,.T.);
#23627=ORIENTED_EDGE('',*,*,#16816,.T.);
#23628=ORIENTED_EDGE('',*,*,#16845,.T.);
#23629=ORIENTED_EDGE('',*,*,#16815,.T.);
#23630=ORIENTED_EDGE('',*,*,#16846,.T.);
#23631=ORIENTED_EDGE('',*,*,#16825,.T.);
#23632=ORIENTED_EDGE('',*,*,#16847,.T.);
#23633=ORIENTED_EDGE('',*,*,#16814,.T.);
#23634=ORIENTED_EDGE('',*,*,#16848,.T.);
#23635=ORIENTED_EDGE('',*,*,#16810,.T.);
#23636=ORIENTED_EDGE('',*,*,#16849,.T.);
#23637=ORIENTED_EDGE('',*,*,#16785,.F.);
#23638=ORIENTED_EDGE('',*,*,#16829,.F.);
#23639=ORIENTED_EDGE('',*,*,#16846,.F.);
#23640=ORIENTED_EDGE('',*,*,#16849,.F.);
#23641=ORIENTED_EDGE('',*,*,#16812,.F.);
#23642=ORIENTED_EDGE('',*,*,#16850,.F.);
#23643=ORIENTED_EDGE('',*,*,#16806,.F.);
#23644=ORIENTED_EDGE('',*,*,#16786,.T.);
#23645=ORIENTED_EDGE('',*,*,#16813,.F.);
#23646=ORIENTED_EDGE('',*,*,#16824,.F.);
#23647=ORIENTED_EDGE('',*,*,#16821,.F.);
#23648=ORIENTED_EDGE('',*,*,#16851,.F.);
#23649=ORIENTED_EDGE('',*,*,#16823,.F.);
#23650=ORIENTED_EDGE('',*,*,#16848,.F.);
#23651=ORIENTED_EDGE('',*,*,#16844,.F.);
#23652=ORIENTED_EDGE('',*,*,#16842,.F.);
#23653=ORIENTED_EDGE('',*,*,#16836,.F.);
#23654=ORIENTED_EDGE('',*,*,#16840,.F.);
#23655=ORIENTED_EDGE('',*,*,#16845,.F.);
#23656=ORIENTED_EDGE('',*,*,#16847,.F.);
#23657=ORIENTED_EDGE('',*,*,#16852,.T.);
#23658=ORIENTED_EDGE('',*,*,#16853,.T.);
#23659=ORIENTED_EDGE('',*,*,#16854,.T.);
#23660=ORIENTED_EDGE('',*,*,#16798,.T.);
#23661=ORIENTED_EDGE('',*,*,#16799,.T.);
#23662=ORIENTED_EDGE('',*,*,#16854,.F.);
#23663=ORIENTED_EDGE('',*,*,#16855,.F.);
#23664=ORIENTED_EDGE('',*,*,#16856,.F.);
#23665=ORIENTED_EDGE('',*,*,#16857,.T.);
#23666=ORIENTED_EDGE('',*,*,#16852,.F.);
#23667=ORIENTED_EDGE('',*,*,#16853,.F.);
#23668=ORIENTED_EDGE('',*,*,#16857,.F.);
#23669=ORIENTED_EDGE('',*,*,#16858,.F.);
#23670=ORIENTED_EDGE('',*,*,#16772,.T.);
#23671=ORIENTED_EDGE('',*,*,#16773,.T.);
#23672=ORIENTED_EDGE('',*,*,#16859,.T.);
#23673=ORIENTED_EDGE('',*,*,#16855,.T.);
#23674=ORIENTED_EDGE('',*,*,#16856,.T.);
#23675=ORIENTED_EDGE('',*,*,#16859,.F.);
#23676=ORIENTED_EDGE('',*,*,#16860,.F.);
#23677=ORIENTED_EDGE('',*,*,#16861,.F.);
#23678=ORIENTED_EDGE('',*,*,#16862,.F.);
#23679=ORIENTED_EDGE('',*,*,#16863,.T.);
#23680=ORIENTED_EDGE('',*,*,#16864,.T.);
#23681=ORIENTED_EDGE('',*,*,#16861,.T.);
#23682=ORIENTED_EDGE('',*,*,#16865,.T.);
#23683=ORIENTED_EDGE('',*,*,#16866,.T.);
#23684=ORIENTED_EDGE('',*,*,#16867,.T.);
#23685=ORIENTED_EDGE('',*,*,#16862,.T.);
#23686=ORIENTED_EDGE('',*,*,#16868,.T.);
#23687=ORIENTED_EDGE('',*,*,#16869,.T.);
#23688=ORIENTED_EDGE('',*,*,#16870,.T.);
#23689=ORIENTED_EDGE('',*,*,#16871,.T.);
#23690=ORIENTED_EDGE('',*,*,#16860,.T.);
#23691=ORIENTED_EDGE('',*,*,#16872,.T.);
#23692=ORIENTED_EDGE('',*,*,#16873,.T.);
#23693=ORIENTED_EDGE('',*,*,#16868,.F.);
#23694=ORIENTED_EDGE('',*,*,#16864,.F.);
#23695=ORIENTED_EDGE('',*,*,#16874,.F.);
#23696=ORIENTED_EDGE('',*,*,#16802,.F.);
#23697=ORIENTED_EDGE('',*,*,#16778,.T.);
#23698=ORIENTED_EDGE('',*,*,#16875,.T.);
#23699=ORIENTED_EDGE('',*,*,#16876,.F.);
#23700=ORIENTED_EDGE('',*,*,#16877,.F.);
#23701=ORIENTED_EDGE('',*,*,#16865,.F.);
#23702=ORIENTED_EDGE('',*,*,#16871,.F.);
#23703=ORIENTED_EDGE('',*,*,#16878,.F.);
#23704=ORIENTED_EDGE('',*,*,#16879,.F.);
#23705=ORIENTED_EDGE('',*,*,#16870,.F.);
#23706=ORIENTED_EDGE('',*,*,#16880,.T.);
#23707=ORIENTED_EDGE('',*,*,#16881,.T.);
#23708=ORIENTED_EDGE('',*,*,#16882,.T.);
#23709=ORIENTED_EDGE('',*,*,#16878,.T.);
#23710=ORIENTED_EDGE('',*,*,#16883,.F.);
#23711=ORIENTED_EDGE('',*,*,#16884,.F.);
#23712=ORIENTED_EDGE('',*,*,#16885,.F.);
#23713=ORIENTED_EDGE('',*,*,#16886,.F.);
#23714=ORIENTED_EDGE('',*,*,#16887,.F.);
#23715=ORIENTED_EDGE('',*,*,#16888,.F.);
#23716=ORIENTED_EDGE('',*,*,#16889,.T.);
#23717=ORIENTED_EDGE('',*,*,#16887,.T.);
#23718=ORIENTED_EDGE('',*,*,#16890,.T.);
#23719=ORIENTED_EDGE('',*,*,#16891,.T.);
#23720=ORIENTED_EDGE('',*,*,#16876,.T.);
#23721=ORIENTED_EDGE('',*,*,#16776,.F.);
#23722=ORIENTED_EDGE('',*,*,#16892,.T.);
#23723=ORIENTED_EDGE('',*,*,#16888,.T.);
#23724=ORIENTED_EDGE('',*,*,#16893,.T.);
#23725=ORIENTED_EDGE('',*,*,#16884,.T.);
#23726=ORIENTED_EDGE('',*,*,#16894,.T.);
#23727=ORIENTED_EDGE('',*,*,#16886,.T.);
#23728=ORIENTED_EDGE('',*,*,#16895,.T.);
#23729=ORIENTED_EDGE('',*,*,#16873,.F.);
#23730=ORIENTED_EDGE('',*,*,#16896,.T.);
#23731=ORIENTED_EDGE('',*,*,#16885,.T.);
#23732=ORIENTED_EDGE('',*,*,#16897,.T.);
#23733=ORIENTED_EDGE('',*,*,#16880,.F.);
#23734=ORIENTED_EDGE('',*,*,#16866,.F.);
#23735=ORIENTED_EDGE('',*,*,#16898,.F.);
#23736=ORIENTED_EDGE('',*,*,#16899,.T.);
#23737=ORIENTED_EDGE('',*,*,#16883,.T.);
#23738=ORIENTED_EDGE('',*,*,#16900,.T.);
#23739=ORIENTED_EDGE('',*,*,#16869,.F.);
#23740=ORIENTED_EDGE('',*,*,#16877,.T.);
#23741=ORIENTED_EDGE('',*,*,#16891,.F.);
#23742=ORIENTED_EDGE('',*,*,#16901,.T.);
#23743=ORIENTED_EDGE('',*,*,#16898,.T.);
#23744=ORIENTED_EDGE('',*,*,#16881,.F.);
#23745=ORIENTED_EDGE('',*,*,#16897,.F.);
#23746=ORIENTED_EDGE('',*,*,#16895,.F.);
#23747=ORIENTED_EDGE('',*,*,#16892,.F.);
#23748=ORIENTED_EDGE('',*,*,#16775,.F.);
#23749=ORIENTED_EDGE('',*,*,#16774,.T.);
#23750=ORIENTED_EDGE('',*,*,#16765,.F.);
#23751=ORIENTED_EDGE('',*,*,#16902,.F.);
#23752=ORIENTED_EDGE('',*,*,#16893,.F.);
#23753=ORIENTED_EDGE('',*,*,#16889,.F.);
#23754=ORIENTED_EDGE('',*,*,#16875,.F.);
#23755=ORIENTED_EDGE('',*,*,#16777,.T.);
#23756=ORIENTED_EDGE('',*,*,#16890,.F.);
#23757=ORIENTED_EDGE('',*,*,#16894,.F.);
#23758=ORIENTED_EDGE('',*,*,#16899,.F.);
#23759=ORIENTED_EDGE('',*,*,#16901,.F.);
#23760=ORIENTED_EDGE('',*,*,#16903,.F.);
#23761=ORIENTED_EDGE('',*,*,#16904,.F.);
#23762=ORIENTED_EDGE('',*,*,#16905,.F.);
#23763=ORIENTED_EDGE('',*,*,#16906,.T.);
#23764=ORIENTED_EDGE('',*,*,#16907,.T.);
#23765=ORIENTED_EDGE('',*,*,#16904,.T.);
#23766=ORIENTED_EDGE('',*,*,#16908,.T.);
#23767=ORIENTED_EDGE('',*,*,#16909,.F.);
#23768=ORIENTED_EDGE('',*,*,#16910,.F.);
#23769=ORIENTED_EDGE('',*,*,#16911,.F.);
#23770=ORIENTED_EDGE('',*,*,#16912,.F.);
#23771=ORIENTED_EDGE('',*,*,#16913,.F.);
#23772=ORIENTED_EDGE('',*,*,#16914,.F.);
#23773=ORIENTED_EDGE('',*,*,#16915,.T.);
#23774=ORIENTED_EDGE('',*,*,#16916,.T.);
#23775=ORIENTED_EDGE('',*,*,#16913,.T.);
#23776=ORIENTED_EDGE('',*,*,#16917,.T.);
#23777=ORIENTED_EDGE('',*,*,#16903,.T.);
#23778=ORIENTED_EDGE('',*,*,#16918,.T.);
#23779=ORIENTED_EDGE('',*,*,#16914,.T.);
#23780=ORIENTED_EDGE('',*,*,#16919,.T.);
#23781=ORIENTED_EDGE('',*,*,#16920,.F.);
#23782=ORIENTED_EDGE('',*,*,#16921,.F.);
#23783=ORIENTED_EDGE('',*,*,#16922,.F.);
#23784=ORIENTED_EDGE('',*,*,#16792,.T.);
#23785=ORIENTED_EDGE('',*,*,#16923,.T.);
#23786=ORIENTED_EDGE('',*,*,#16921,.T.);
#23787=ORIENTED_EDGE('',*,*,#16924,.T.);
#23788=ORIENTED_EDGE('',*,*,#16925,.F.);
#23789=ORIENTED_EDGE('',*,*,#16926,.F.);
#23790=ORIENTED_EDGE('',*,*,#16927,.F.);
#23791=ORIENTED_EDGE('',*,*,#16928,.F.);
#23792=ORIENTED_EDGE('',*,*,#16929,.F.);
#23793=ORIENTED_EDGE('',*,*,#16930,.F.);
#23794=ORIENTED_EDGE('',*,*,#16929,.T.);
#23795=ORIENTED_EDGE('',*,*,#16931,.T.);
#23796=ORIENTED_EDGE('',*,*,#16922,.T.);
#23797=ORIENTED_EDGE('',*,*,#16932,.T.);
#23798=ORIENTED_EDGE('',*,*,#16790,.F.);
#23799=ORIENTED_EDGE('',*,*,#16933,.T.);
#23800=ORIENTED_EDGE('',*,*,#16930,.T.);
#23801=ORIENTED_EDGE('',*,*,#16934,.T.);
#23802=ORIENTED_EDGE('',*,*,#16926,.T.);
#23803=ORIENTED_EDGE('',*,*,#16935,.T.);
#23804=ORIENTED_EDGE('',*,*,#16928,.T.);
#23805=ORIENTED_EDGE('',*,*,#16936,.T.);
#23806=ORIENTED_EDGE('',*,*,#16912,.T.);
#23807=ORIENTED_EDGE('',*,*,#16937,.T.);
#23808=ORIENTED_EDGE('',*,*,#16927,.T.);
#23809=ORIENTED_EDGE('',*,*,#16938,.T.);
#23810=ORIENTED_EDGE('',*,*,#16925,.T.);
#23811=ORIENTED_EDGE('',*,*,#16939,.T.);
#23812=ORIENTED_EDGE('',*,*,#16911,.T.);
#23813=ORIENTED_EDGE('',*,*,#16940,.T.);
#23814=ORIENTED_EDGE('',*,*,#16910,.T.);
#23815=ORIENTED_EDGE('',*,*,#16941,.T.);
#23816=ORIENTED_EDGE('',*,*,#16920,.T.);
#23817=ORIENTED_EDGE('',*,*,#16942,.T.);
#23818=ORIENTED_EDGE('',*,*,#16909,.T.);
#23819=ORIENTED_EDGE('',*,*,#16943,.T.);
#23820=ORIENTED_EDGE('',*,*,#16905,.T.);
#23821=ORIENTED_EDGE('',*,*,#16944,.T.);
#23822=ORIENTED_EDGE('',*,*,#16793,.F.);
#23823=ORIENTED_EDGE('',*,*,#16924,.F.);
#23824=ORIENTED_EDGE('',*,*,#16941,.F.);
#23825=ORIENTED_EDGE('',*,*,#16944,.F.);
#23826=ORIENTED_EDGE('',*,*,#16907,.F.);
#23827=ORIENTED_EDGE('',*,*,#16945,.F.);
#23828=ORIENTED_EDGE('',*,*,#16768,.F.);
#23829=ORIENTED_EDGE('',*,*,#16770,.T.);
#23830=ORIENTED_EDGE('',*,*,#16908,.F.);
#23831=ORIENTED_EDGE('',*,*,#16919,.F.);
#23832=ORIENTED_EDGE('',*,*,#16916,.F.);
#23833=ORIENTED_EDGE('',*,*,#16946,.F.);
#23834=ORIENTED_EDGE('',*,*,#16918,.F.);
#23835=ORIENTED_EDGE('',*,*,#16943,.F.);
#23836=ORIENTED_EDGE('',*,*,#16939,.F.);
#23837=ORIENTED_EDGE('',*,*,#16937,.F.);
#23838=ORIENTED_EDGE('',*,*,#16931,.F.);
#23839=ORIENTED_EDGE('',*,*,#16935,.F.);
#23840=ORIENTED_EDGE('',*,*,#16940,.F.);
#23841=ORIENTED_EDGE('',*,*,#16942,.F.);
#23842=ORIENTED_EDGE('',*,*,#16947,.T.);
#23843=ORIENTED_EDGE('',*,*,#16948,.T.);
#23844=ORIENTED_EDGE('',*,*,#16947,.F.);
#23845=ORIENTED_EDGE('',*,*,#16858,.T.);
#23846=ORIENTED_EDGE('',*,*,#16948,.F.);
#23847=ORIENTED_EDGE('',*,*,#16949,.T.);
#23848=ORIENTED_EDGE('',*,*,#16950,.T.);
#23849=ORIENTED_EDGE('',*,*,#16951,.T.);
#23850=ORIENTED_EDGE('',*,*,#16949,.F.);
#23851=ORIENTED_EDGE('',*,*,#16952,.T.);
#23852=ORIENTED_EDGE('',*,*,#16951,.F.);
#23853=ORIENTED_EDGE('',*,*,#16953,.F.);
#23854=ORIENTED_EDGE('',*,*,#16950,.F.);
#23855=ORIENTED_EDGE('',*,*,#16789,.F.);
#23856=ORIENTED_EDGE('',*,*,#16788,.T.);
#23857=ORIENTED_EDGE('',*,*,#16805,.F.);
#23858=ORIENTED_EDGE('',*,*,#16954,.F.);
#23859=ORIENTED_EDGE('',*,*,#16917,.F.);
#23860=ORIENTED_EDGE('',*,*,#16938,.F.);
#23861=ORIENTED_EDGE('',*,*,#16936,.F.);
#23862=ORIENTED_EDGE('',*,*,#16933,.F.);
#23863=ORIENTED_EDGE('',*,*,#16923,.F.);
#23864=ORIENTED_EDGE('',*,*,#16791,.T.);
#23865=ORIENTED_EDGE('',*,*,#16934,.F.);
#23866=ORIENTED_EDGE('',*,*,#16932,.F.);
#23867=ORIENTED_EDGE('',*,*,#16867,.F.);
#23868=ORIENTED_EDGE('',*,*,#16900,.F.);
#23869=ORIENTED_EDGE('',*,*,#16896,.F.);
#23870=ORIENTED_EDGE('',*,*,#16872,.F.);
#23871=ORIENTED_EDGE('',*,*,#16781,.F.);
#23872=ORIENTED_EDGE('',*,*,#16780,.T.);
#23873=ORIENTED_EDGE('',*,*,#16804,.F.);
#23874=ORIENTED_EDGE('',*,*,#16955,.F.);
#23875=ORIENTED_EDGE('',*,*,#16822,.F.);
#23876=ORIENTED_EDGE('',*,*,#16843,.F.);
#23877=ORIENTED_EDGE('',*,*,#16841,.F.);
#23878=ORIENTED_EDGE('',*,*,#16838,.F.);
#23879=ORIENTED_EDGE('',*,*,#16828,.F.);
#23880=ORIENTED_EDGE('',*,*,#16783,.T.);
#23881=ORIENTED_EDGE('',*,*,#16839,.F.);
#23882=ORIENTED_EDGE('',*,*,#16837,.F.);
#23883=ORIENTED_EDGE('',*,*,#16956,.T.);
#23884=ORIENTED_EDGE('',*,*,#16957,.T.);
#23885=ORIENTED_EDGE('',*,*,#16953,.T.);
#23886=ORIENTED_EDGE('',*,*,#16958,.T.);
#23887=ORIENTED_EDGE('',*,*,#16801,.F.);
#23888=ORIENTED_EDGE('',*,*,#16958,.F.);
#23889=ORIENTED_EDGE('',*,*,#16952,.F.);
#23890=ORIENTED_EDGE('',*,*,#16957,.F.);
#23891=ORIENTED_EDGE('',*,*,#16769,.F.);
#23892=ORIENTED_EDGE('',*,*,#16945,.T.);
#23893=ORIENTED_EDGE('',*,*,#16906,.F.);
#23894=ORIENTED_EDGE('',*,*,#16946,.T.);
#23895=ORIENTED_EDGE('',*,*,#16915,.F.);
#23896=ORIENTED_EDGE('',*,*,#16954,.T.);
#23897=ORIENTED_EDGE('',*,*,#16807,.F.);
#23898=ORIENTED_EDGE('',*,*,#16850,.T.);
#23899=ORIENTED_EDGE('',*,*,#16811,.F.);
#23900=ORIENTED_EDGE('',*,*,#16851,.T.);
#23901=ORIENTED_EDGE('',*,*,#16820,.F.);
#23902=ORIENTED_EDGE('',*,*,#16955,.T.);
#23903=ORIENTED_EDGE('',*,*,#16803,.F.);
#23904=ORIENTED_EDGE('',*,*,#16874,.T.);
#23905=ORIENTED_EDGE('',*,*,#16863,.F.);
#23906=ORIENTED_EDGE('',*,*,#16879,.T.);
#23907=ORIENTED_EDGE('',*,*,#16882,.F.);
#23908=ORIENTED_EDGE('',*,*,#16902,.T.);
#23909=ORIENTED_EDGE('',*,*,#16956,.F.);
#26799=ADVANCED_FACE('',(#7975),#398,.T.);
#26800=ADVANCED_FACE('',(#7976),#399,.T.);
#26801=ADVANCED_FACE('',(#7977),#400,.T.);
#26802=ADVANCED_FACE('',(#7978),#401,.T.);
#26803=ADVANCED_FACE('',(#7979,#713),#1474,.T.);
#26804=ADVANCED_FACE('',(#7980),#402,.T.);
#26805=ADVANCED_FACE('',(#7981),#403,.T.);
#26806=ADVANCED_FACE('',(#7982),#1475,.T.);
#26807=ADVANCED_FACE('',(#7983),#1476,.T.);
#26808=ADVANCED_FACE('',(#7984),#1477,.T.);
#26809=ADVANCED_FACE('',(#7985),#1478,.T.);
#26810=ADVANCED_FACE('',(#7986),#1479,.T.);
#26811=ADVANCED_FACE('',(#7987),#1480,.T.);
#26812=ADVANCED_FACE('',(#7988),#1481,.T.);
#26813=ADVANCED_FACE('',(#7989),#1482,.T.);
#26814=ADVANCED_FACE('',(#7990),#1483,.T.);
#26815=ADVANCED_FACE('',(#7991),#1484,.T.);
#26816=ADVANCED_FACE('',(#7992),#1485,.T.);
#26817=ADVANCED_FACE('',(#7993),#1486,.T.);
#26818=ADVANCED_FACE('',(#7994),#1487,.T.);
#26819=ADVANCED_FACE('',(#7995),#1488,.T.);
#26820=ADVANCED_FACE('',(#7996),#1489,.T.);
#26821=ADVANCED_FACE('',(#7997),#1490,.T.);
#26822=ADVANCED_FACE('',(#7998),#1491,.T.);
#26823=ADVANCED_FACE('',(#7999),#1492,.T.);
#26824=ADVANCED_FACE('',(#8000),#1493,.T.);
#26825=ADVANCED_FACE('',(#8001),#1494,.T.);
#26826=ADVANCED_FACE('',(#8002),#1495,.T.);
#26827=ADVANCED_FACE('',(#8003),#404,.T.);
#26828=ADVANCED_FACE('',(#8004,#714),#6711,.T.);
#26829=ADVANCED_FACE('',(#8005),#405,.T.);
#26830=ADVANCED_FACE('',(#8006),#1496,.T.);
#26831=ADVANCED_FACE('',(#8007),#1497,.T.);
#26832=ADVANCED_FACE('',(#8008),#1498,.T.);
#26833=ADVANCED_FACE('',(#8009),#1499,.T.);
#26834=ADVANCED_FACE('',(#8010),#1500,.T.);
#26835=ADVANCED_FACE('',(#8011),#1501,.T.);
#26836=ADVANCED_FACE('',(#8012),#1502,.T.);
#26837=ADVANCED_FACE('',(#8013),#1503,.T.);
#26838=ADVANCED_FACE('',(#8014),#1504,.T.);
#26839=ADVANCED_FACE('',(#8015),#1505,.T.);
#26840=ADVANCED_FACE('',(#8016),#1506,.T.);
#26841=ADVANCED_FACE('',(#8017),#1507,.T.);
#26842=ADVANCED_FACE('',(#8018),#1508,.T.);
#26843=ADVANCED_FACE('',(#8019),#1509,.T.);
#26844=ADVANCED_FACE('',(#8020),#1510,.T.);
#26845=ADVANCED_FACE('',(#8021),#1511,.T.);
#26846=ADVANCED_FACE('',(#8022),#1512,.F.);
#26847=ADVANCED_FACE('',(#8023),#1513,.T.);
#26848=ADVANCED_FACE('',(#8024),#1514,.T.);
#26849=ADVANCED_FACE('',(#8025),#1515,.T.);
#26850=ADVANCED_FACE('',(#8026),#1516,.T.);
#26851=ADVANCED_FACE('',(#8027),#1517,.T.);
#26852=ADVANCED_FACE('',(#8028),#1518,.T.);
#26853=ADVANCED_FACE('',(#8029),#1519,.T.);
#26854=ADVANCED_FACE('',(#8030),#1520,.T.);
#26855=ADVANCED_FACE('',(#8031),#1521,.T.);
#26856=ADVANCED_FACE('',(#8032),#1522,.T.);
#26857=ADVANCED_FACE('',(#8033),#1523,.T.);
#26858=ADVANCED_FACE('',(#8034),#1524,.T.);
#26859=ADVANCED_FACE('',(#8035),#1525,.T.);
#26860=ADVANCED_FACE('',(#8036),#1526,.T.);
#26861=ADVANCED_FACE('',(#8037),#1527,.T.);
#26862=ADVANCED_FACE('',(#8038),#1528,.T.);
#26863=ADVANCED_FACE('',(#8039),#1529,.T.);
#26864=ADVANCED_FACE('',(#8040),#1530,.T.);
#26865=ADVANCED_FACE('',(#8041),#1531,.T.);
#26866=ADVANCED_FACE('',(#8042),#1532,.T.);
#26867=ADVANCED_FACE('',(#8043),#1533,.T.);
#26868=ADVANCED_FACE('',(#8044),#1534,.T.);
#26869=ADVANCED_FACE('',(#8045),#577,.T.);
#26870=ADVANCED_FACE('',(#8046),#6712,.F.);
#26871=ADVANCED_FACE('',(#8047),#1535,.T.);
#26872=ADVANCED_FACE('',(#8048),#1536,.T.);
#26873=ADVANCED_FACE('',(#8049),#1537,.T.);
#26874=ADVANCED_FACE('',(#8050),#1538,.F.);
#26875=ADVANCED_FACE('',(#8051),#1539,.T.);
#26876=ADVANCED_FACE('',(#8052),#1540,.T.);
#26877=ADVANCED_FACE('',(#8053),#1541,.F.);
#26878=ADVANCED_FACE('',(#8054),#6713,.F.);
#26879=ADVANCED_FACE('',(#8055,#715),#1542,.T.);
#27236=CLOSED_SHELL('',(#26799,#26800,#26801,#26802,#26803,#26804,#26805,
#26806,#26807,#26808,#26809,#26810,#26811,#26812,#26813,#26814,#26815,#26816,
#26817,#26818,#26819,#26820,#26821,#26822,#26823,#26824,#26825,#26826,#26827,
#26828,#26829,#26830,#26831,#26832,#26833,#26834,#26835,#26836,#26837,#26838,
#26839,#26840,#26841,#26842,#26843,#26844,#26845,#26846,#26847,#26848,#26849,
#26850,#26851,#26852,#26853,#26854,#26855,#26856,#26857,#26858,#26859,#26860,
#26861,#26862,#26863,#26864,#26865,#26866,#26867,#26868,#26869,#26870,#26871,
#26872,#26873,#26874,#26875,#26876,#26877,#26878,#26879));
#29390=AXIS2_PLACEMENT_3D('',#46089,#35566,#35567);
#29391=AXIS2_PLACEMENT_3D('',#46090,#35568,#35569);
#29392=AXIS2_PLACEMENT_3D('',#46097,#35570,#35571);
#29393=AXIS2_PLACEMENT_3D('',#46099,#35572,#35573);
#29394=AXIS2_PLACEMENT_3D('',#46104,#35574,#35575);
#29395=AXIS2_PLACEMENT_3D('',#46105,#35576,#35577);
#29396=AXIS2_PLACEMENT_3D('',#46113,#35579,#35580);
#29397=AXIS2_PLACEMENT_3D('',#46114,#35581,#35582);
#29398=AXIS2_PLACEMENT_3D('',#46128,#35583,#35584);
#29399=AXIS2_PLACEMENT_3D('',#46134,#35585,#35586);
#29400=AXIS2_PLACEMENT_3D('',#46148,#35587,#35588);
#29401=AXIS2_PLACEMENT_3D('',#46162,#35589,#35590);
#29402=AXIS2_PLACEMENT_3D('',#46176,#35591,#35592);
#29403=AXIS2_PLACEMENT_3D('',#46184,#35593,#35594);
#29404=AXIS2_PLACEMENT_3D('',#46187,#35595,#35596);
#29405=AXIS2_PLACEMENT_3D('',#46188,#35597,#35598);
#29406=AXIS2_PLACEMENT_3D('',#46191,#35600,#35601);
#29407=AXIS2_PLACEMENT_3D('',#46192,#35602,#35603);
#29408=AXIS2_PLACEMENT_3D('',#46195,#35604,#35605);
#29409=AXIS2_PLACEMENT_3D('',#46196,#35606,#35607);
#29410=AXIS2_PLACEMENT_3D('',#46198,#35609,#35610);
#29411=AXIS2_PLACEMENT_3D('',#46200,#35611,#35612);
#29412=AXIS2_PLACEMENT_3D('',#46201,#35613,#35614);
#29413=AXIS2_PLACEMENT_3D('',#46207,#35615,#35616);
#29414=AXIS2_PLACEMENT_3D('',#46211,#35617,#35618);
#29415=AXIS2_PLACEMENT_3D('',#46220,#35619,#35620);
#29416=AXIS2_PLACEMENT_3D('',#46221,#35621,#35622);
#29417=AXIS2_PLACEMENT_3D('',#46228,#35626,#35627);
#29418=AXIS2_PLACEMENT_3D('',#46234,#35631,#35632);
#29419=AXIS2_PLACEMENT_3D('',#46241,#35636,#35637);
#29420=AXIS2_PLACEMENT_3D('',#46248,#35641,#35642);
#29421=AXIS2_PLACEMENT_3D('',#46254,#35646,#35647);
#29422=AXIS2_PLACEMENT_3D('',#46257,#35650,#35651);
#29423=AXIS2_PLACEMENT_3D('',#46264,#35655,#35656);
#29424=AXIS2_PLACEMENT_3D('',#46267,#35659,#35660);
#29425=AXIS2_PLACEMENT_3D('',#46274,#35664,#35665);
#29426=AXIS2_PLACEMENT_3D('',#46281,#35669,#35670);
#29427=AXIS2_PLACEMENT_3D('',#46284,#35673,#35674);
#29428=AXIS2_PLACEMENT_3D('',#46287,#35677,#35678);
#29429=AXIS2_PLACEMENT_3D('',#46290,#35681,#35682);
#29430=AXIS2_PLACEMENT_3D('',#46293,#35685,#35686);
#29431=AXIS2_PLACEMENT_3D('',#46296,#35689,#35690);
#29432=AXIS2_PLACEMENT_3D('',#46299,#35693,#35694);
#29433=AXIS2_PLACEMENT_3D('',#46302,#35697,#35698);
#29434=AXIS2_PLACEMENT_3D('',#46304,#35700,#35701);
#29435=AXIS2_PLACEMENT_3D('',#46306,#35703,#35704);
#29436=AXIS2_PLACEMENT_3D('',#46307,#35705,#35706);
#29437=AXIS2_PLACEMENT_3D('',#46308,#35707,#35708);
#29438=AXIS2_PLACEMENT_3D('',#46311,#35709,#35710);
#29439=AXIS2_PLACEMENT_3D('',#46312,#35711,#35712);
#29440=AXIS2_PLACEMENT_3D('',#46314,#35714,#35715);
#29441=AXIS2_PLACEMENT_3D('',#46317,#35716,#35717);
#29442=AXIS2_PLACEMENT_3D('',#46318,#35718,#35719);
#29443=AXIS2_PLACEMENT_3D('',#46351,#35721,#35722);
#29444=AXIS2_PLACEMENT_3D('',#46353,#35724,#35725);
#29445=AXIS2_PLACEMENT_3D('',#46360,#35729,#35730);
#29446=AXIS2_PLACEMENT_3D('',#46366,#35734,#35735);
#29447=AXIS2_PLACEMENT_3D('',#46374,#35740,#35741);
#29448=AXIS2_PLACEMENT_3D('',#46382,#35746,#35747);
#29449=AXIS2_PLACEMENT_3D('',#46389,#35752,#35753);
#29450=AXIS2_PLACEMENT_3D('',#46393,#35756,#35757);
#29451=AXIS2_PLACEMENT_3D('',#46399,#35761,#35762);
#29452=AXIS2_PLACEMENT_3D('',#46406,#35766,#35767);
#29453=AXIS2_PLACEMENT_3D('',#46413,#35771,#35772);
#29454=AXIS2_PLACEMENT_3D('',#46418,#35776,#35777);
#29455=AXIS2_PLACEMENT_3D('',#46421,#35780,#35781);
#29456=AXIS2_PLACEMENT_3D('',#46424,#35784,#35785);
#29457=AXIS2_PLACEMENT_3D('',#46427,#35788,#35789);
#29458=AXIS2_PLACEMENT_3D('',#46432,#35793,#35794);
#29459=AXIS2_PLACEMENT_3D('',#46434,#35796,#35797);
#29460=AXIS2_PLACEMENT_3D('',#46436,#35799,#35800);
#29461=AXIS2_PLACEMENT_3D('',#46437,#35801,#35802);
#29462=AXIS2_PLACEMENT_3D('',#46438,#35803,#35804);
#29463=AXIS2_PLACEMENT_3D('',#46445,#35808,#35809);
#29464=AXIS2_PLACEMENT_3D('',#46451,#35813,#35814);
#29465=AXIS2_PLACEMENT_3D('',#46458,#35818,#35819);
#29466=AXIS2_PLACEMENT_3D('',#46465,#35823,#35824);
#29467=AXIS2_PLACEMENT_3D('',#46471,#35828,#35829);
#29468=AXIS2_PLACEMENT_3D('',#46474,#35832,#35833);
#29469=AXIS2_PLACEMENT_3D('',#46481,#35837,#35838);
#29470=AXIS2_PLACEMENT_3D('',#46484,#35841,#35842);
#29471=AXIS2_PLACEMENT_3D('',#46491,#35846,#35847);
#29472=AXIS2_PLACEMENT_3D('',#46498,#35851,#35852);
#29473=AXIS2_PLACEMENT_3D('',#46501,#35855,#35856);
#29474=AXIS2_PLACEMENT_3D('',#46504,#35859,#35860);
#29475=AXIS2_PLACEMENT_3D('',#46507,#35863,#35864);
#29476=AXIS2_PLACEMENT_3D('',#46510,#35867,#35868);
#29477=AXIS2_PLACEMENT_3D('',#46513,#35871,#35872);
#29478=AXIS2_PLACEMENT_3D('',#46516,#35875,#35876);
#29479=AXIS2_PLACEMENT_3D('',#46519,#35879,#35880);
#29480=AXIS2_PLACEMENT_3D('',#46521,#35882,#35883);
#29481=AXIS2_PLACEMENT_3D('',#46523,#35885,#35886);
#29482=AXIS2_PLACEMENT_3D('',#46524,#35887,#35888);
#29483=AXIS2_PLACEMENT_3D('',#46677,#35890,#35891);
#29484=AXIS2_PLACEMENT_3D('',#46681,#35893,#35894);
#29485=AXIS2_PLACEMENT_3D('',#46682,#35895,#35896);
#29486=AXIS2_PLACEMENT_3D('',#46683,#35897,#35898);
#29487=AXIS2_PLACEMENT_3D('',#46685,#35900,#35901);
#29488=AXIS2_PLACEMENT_3D('',#46687,#35903,#35904);
#29489=AXIS2_PLACEMENT_3D('',#46689,#35906,#35907);
#29490=AXIS2_PLACEMENT_3D('',#46690,#35908,#35909);
#29491=AXIS2_PLACEMENT_3D('',#46691,#35910,#35911);
#29492=AXIS2_PLACEMENT_3D('',#46693,#35913,#35914);
#29493=AXIS2_PLACEMENT_3D('',#46694,#35915,#35916);
#29494=AXIS2_PLACEMENT_3D('',#46696,#35917,#35918);
#29495=AXIS2_PLACEMENT_3D('',#46699,#35921,#35922);
#35566=DIRECTION('axis',(0.,0.,1.));
#35567=DIRECTION('refdir',(1.,0.,0.));
#35568=DIRECTION('center_axis',(-1.,0.,-4.21782140988753E-15));
#35569=DIRECTION('ref_axis',(0.,-1.,-3.1162263922408E-17));
#35570=DIRECTION('center_axis',(1.,0.,0.));
#35571=DIRECTION('ref_axis',(0.,-1.,-6.12323399573677E-17));
#35572=DIRECTION('center_axis',(1.,0.,0.));
#35573=DIRECTION('ref_axis',(0.,-1.,-6.12323399573677E-17));
#35574=DIRECTION('center_axis',(-1.,0.,0.));
#35575=DIRECTION('ref_axis',(0.,-1.,0.));
#35576=DIRECTION('center_axis',(-1.,0.,0.));
#35577=DIRECTION('ref_axis',(0.,1.,0.));
#35578=DIRECTION('',(-0.707106781186552,-0.707106781186543,-8.65956056235487E-17));
#35579=DIRECTION('center_axis',(-1.,0.,0.));
#35580=DIRECTION('ref_axis',(0.,-1.,-6.12323399573676E-17));
#35581=DIRECTION('center_axis',(-1.,0.,0.));
#35582=DIRECTION('ref_axis',(0.,-1.,-6.12323399573676E-17));
#35583=DIRECTION('center_axis',(1.,0.,0.));
#35584=DIRECTION('ref_axis',(0.,0.,-1.));
#35585=DIRECTION('center_axis',(1.,0.,0.));
#35586=DIRECTION('ref_axis',(0.,1.,6.12323399573677E-17));
#35587=DIRECTION('center_axis',(1.,0.,0.));
#35588=DIRECTION('ref_axis',(0.,0.,-1.));
#35589=DIRECTION('center_axis',(1.,0.,0.));
#35590=DIRECTION('ref_axis',(0.,1.,6.12323399573677E-17));
#35591=DIRECTION('center_axis',(1.,0.,0.));
#35592=DIRECTION('ref_axis',(0.,0.,-1.));
#35593=DIRECTION('center_axis',(1.,0.,-4.21782140988753E-15));
#35594=DIRECTION('ref_axis',(0.,-1.,-3.1162263922408E-17));
#35595=DIRECTION('center_axis',(-1.,0.,0.));
#35596=DIRECTION('ref_axis',(0.,-1.,-6.12323399573677E-17));
#35597=DIRECTION('center_axis',(-1.,0.,0.));
#35598=DIRECTION('ref_axis',(0.,-1.,-6.12323399573677E-17));
#35599=DIRECTION('',(-0.382683432365103,-0.923879532511281,1.47215758518538E-15));
#35600=DIRECTION('center_axis',(1.,0.,0.));
#35601=DIRECTION('ref_axis',(0.,-1.,0.));
#35602=DIRECTION('center_axis',(1.,0.,0.));
#35603=DIRECTION('ref_axis',(0.,1.,0.));
#35604=DIRECTION('center_axis',(1.,0.,0.));
#35605=DIRECTION('ref_axis',(0.,-1.,-6.12323399573676E-17));
#35606=DIRECTION('center_axis',(1.,0.,0.));
#35607=DIRECTION('ref_axis',(0.,-1.,-6.12323399573676E-17));
#35608=DIRECTION('',(-0.707106781186552,0.707106781186543,8.65956056235487E-17));
#35609=DIRECTION('center_axis',(-1.,0.,0.));
#35610=DIRECTION('ref_axis',(0.,0.,1.));
#35611=DIRECTION('center_axis',(1.,0.,0.));
#35612=DIRECTION('ref_axis',(0.,0.,-1.));
#35613=DIRECTION('center_axis',(-1.,0.,-4.21782140988753E-15));
#35614=DIRECTION('ref_axis',(0.,1.,3.1162263922408E-17));
#35615=DIRECTION('center_axis',(-1.,0.,0.));
#35616=DIRECTION('ref_axis',(0.,1.,0.));
#35617=DIRECTION('center_axis',(-1.,0.,-4.21782140988753E-15));
#35618=DIRECTION('ref_axis',(0.,1.,3.1162263922408E-17));
#35619=DIRECTION('center_axis',(-1.,0.,0.));
#35620=DIRECTION('ref_axis',(0.,1.,0.));
#35621=DIRECTION('center_axis',(0.553280795424863,-0.635591688956665,-0.538426936866317));
#35622=DIRECTION('ref_axis',(-0.697421280285469,0.,-0.716661396898826));
#35623=DIRECTION('',(0.703011344182424,0.703011344182365,-0.107471391084913));
#35624=DIRECTION('',(0.,-0.646374896130196,0.763019982472725));
#35625=DIRECTION('',(-0.703011344182424,-0.00956522589581351,-0.71111430614521));
#35626=DIRECTION('center_axis',(0.,-0.763019982472725,-0.646374896130196));
#35627=DIRECTION('ref_axis',(-1.,0.,0.));
#35628=DIRECTION('',(0.,-0.646374896130196,0.763019982472725));
#35629=DIRECTION('',(1.,0.,0.));
#35630=DIRECTION('',(-1.,0.,0.));
#35631=DIRECTION('center_axis',(0.61702108254174,0.508662540160709,-0.600455996669427));
#35632=DIRECTION('ref_axis',(-0.697421280285471,0.,-0.716661396898825));
#35633=DIRECTION('',(0.701419241812877,-0.0095435636297033,0.712685040959816));
#35634=DIRECTION('',(0.,-0.763019982472724,-0.646374896130198));
#35635=DIRECTION('',(-0.701419241812879,0.701419241812816,-0.126578412177515));
#35636=DIRECTION('center_axis',(0.553280795424862,-0.635591688956666,0.538426936866317));
#35637=DIRECTION('ref_axis',(0.69742128028547,0.,-0.716661396898825));
#35638=DIRECTION('',(0.703011344182427,0.00956522589581354,-0.711114306145207));
#35639=DIRECTION('',(0.,0.646374896130195,0.763019982472726));
#35640=DIRECTION('',(-0.703011344182424,-0.703011344182364,-0.107471391084915));
#35641=DIRECTION('center_axis',(0.,-0.763019982472726,0.646374896130195));
#35642=DIRECTION('ref_axis',(1.,0.,0.));
#35643=DIRECTION('',(0.,0.646374896130195,0.763019982472726));
#35644=DIRECTION('',(1.,0.,0.));
#35645=DIRECTION('',(-1.,0.,0.));
#35646=DIRECTION('center_axis',(0.707106781186518,-0.707106781186577,0.));
#35647=DIRECTION('ref_axis',(0.,0.,-1.));
#35648=DIRECTION('',(0.,0.,1.));
#35649=DIRECTION('',(0.,0.,-1.));
#35650=DIRECTION('center_axis',(-0.617021082541767,0.508662540160695,-0.60045599666941));
#35651=DIRECTION('ref_axis',(-0.697421280285445,0.,0.71666139689885));
#35652=DIRECTION('',(0.,0.763019982472724,0.646374896130198));
#35653=DIRECTION('',(0.701419241812852,0.00954356362970364,-0.712685040959841));
#35654=DIRECTION('',(-0.701419241812853,-0.701419241812841,0.12657841217752));
#35655=DIRECTION('center_axis',(-0.707106781186542,-0.11624763874382,-0.697485832462921));
#35656=DIRECTION('ref_axis',(-0.702246883176789,0.,0.711933504667737));
#35657=DIRECTION('',(0.,0.986393923832144,-0.164398987305357));
#35658=DIRECTION('',(0.,-0.986393923832144,0.164398987305357));
#35659=DIRECTION('center_axis',(0.617021082541738,0.508662540160709,0.600455996669429));
#35660=DIRECTION('ref_axis',(0.697421280285473,0.,-0.716661396898823));
#35661=DIRECTION('',(0.701419241812879,-0.701419241812817,-0.126578412177511));
#35662=DIRECTION('',(0.,0.763019982472725,-0.646374896130197));
#35663=DIRECTION('',(-0.701419241812879,0.00954356362970333,0.712685040959814));
#35664=DIRECTION('center_axis',(-0.617021082541767,0.508662540160693,0.600455996669412));
#35665=DIRECTION('ref_axis',(0.697421280285446,0.,0.716661396898849));
#35666=DIRECTION('',(0.,-0.763019982472725,0.646374896130197));
#35667=DIRECTION('',(0.701419241812853,0.701419241812841,0.126578412177521));
#35668=DIRECTION('',(-0.701419241812852,-0.00954356362970365,-0.71268504095984));
#35669=DIRECTION('center_axis',(-0.707106781186541,0.707106781186554,0.));
#35670=DIRECTION('ref_axis',(0.,0.,1.));
#35671=DIRECTION('',(0.,0.,-1.));
#35672=DIRECTION('',(0.,0.,1.));
#35673=DIRECTION('center_axis',(-0.707106781186542,-0.11624763874382,0.697485832462921));
#35674=DIRECTION('ref_axis',(0.702246883176789,0.,0.711933504667736));
#35675=DIRECTION('',(0.,0.986393923832144,0.164398987305357));
#35676=DIRECTION('',(0.,-0.986393923832144,-0.164398987305357));
#35677=DIRECTION('center_axis',(0.,0.646374896130197,0.763019982472725));
#35678=DIRECTION('ref_axis',(1.,0.,0.));
#35679=DIRECTION('',(-1.,0.,0.));
#35680=DIRECTION('',(1.,0.,0.));
#35681=DIRECTION('center_axis',(0.707106781186515,-0.116247638743825,0.697485832462947));
#35682=DIRECTION('ref_axis',(0.702246883176816,0.,-0.71193350466771));
#35683=DIRECTION('',(0.,0.986393923832144,0.164398987305357));
#35684=DIRECTION('',(0.,-0.986393923832144,-0.164398987305357));
#35685=DIRECTION('center_axis',(0.707106781186516,0.707106781186579,0.));
#35686=DIRECTION('ref_axis',(0.,0.,-1.));
#35687=DIRECTION('',(0.,0.,-1.));
#35688=DIRECTION('',(0.,0.,1.));
#35689=DIRECTION('center_axis',(0.,0.646374896130198,-0.763019982472724));
#35690=DIRECTION('ref_axis',(-1.,0.,0.));
#35691=DIRECTION('',(-1.,0.,0.));
#35692=DIRECTION('',(1.,0.,0.));
#35693=DIRECTION('center_axis',(0.707106781186517,-0.116247638743824,-0.697485832462946));
#35694=DIRECTION('ref_axis',(-0.702246883176814,0.,-0.711933504667711));
#35695=DIRECTION('',(0.,-0.986393923832144,0.164398987305357));
#35696=DIRECTION('',(0.,0.986393923832144,-0.164398987305357));
#35697=DIRECTION('center_axis',(0.,-0.164398987305357,-0.986393923832144));
#35698=DIRECTION('ref_axis',(0.,0.986393923832144,-0.164398987305357));
#35699=DIRECTION('',(0.,-0.986393923832144,0.164398987305357));
#35700=DIRECTION('center_axis',(0.,-1.,0.));
#35701=DIRECTION('ref_axis',(0.,0.,-1.));
#35702=DIRECTION('',(0.,0.,1.));
#35703=DIRECTION('center_axis',(1.,0.,0.));
#35704=DIRECTION('ref_axis',(0.,0.,-1.));
#35705=DIRECTION('center_axis',(0.,1.,0.));
#35706=DIRECTION('ref_axis',(0.,0.,1.));
#35707=DIRECTION('center_axis',(1.,0.,1.76809044889307E-15));
#35708=DIRECTION('ref_axis',(0.,-1.,-3.03981392545898E-17));
#35709=DIRECTION('center_axis',(-1.,0.,0.));
#35710=DIRECTION('ref_axis',(0.,-1.,0.));
#35711=DIRECTION('center_axis',(-1.,0.,0.));
#35712=DIRECTION('ref_axis',(0.,-1.,0.));
#35713=DIRECTION('',(-0.923879532511294,-0.382683432365072,-1.69200064568173E-15));
#35714=DIRECTION('center_axis',(1.,0.,0.));
#35715=DIRECTION('ref_axis',(0.,1.,0.));
#35716=DIRECTION('center_axis',(1.,0.,0.));
#35717=DIRECTION('ref_axis',(0.,-1.,0.));
#35718=DIRECTION('center_axis',(1.,0.,0.));
#35719=DIRECTION('ref_axis',(0.,-1.,0.));
#35720=DIRECTION('',(-1.,0.,0.));
#35721=DIRECTION('center_axis',(-1.,0.,1.76809044889307E-15));
#35722=DIRECTION('ref_axis',(0.,-1.,-3.03981392545898E-17));
#35723=DIRECTION('',(-0.923879532511294,0.382683432365072,1.69200064568173E-15));
#35724=DIRECTION('center_axis',(0.553280795424864,0.784087249886401,-0.281225080637575));
#35725=DIRECTION('ref_axis',(-0.453113352871865,0.,-0.891452909271834));
#35726=DIRECTION('',(0.703011344182424,-0.258432717231594,0.66256137875303));
#35727=DIRECTION('',(0.,-0.337607240351444,-0.941287071653639));
#35728=DIRECTION('',(-0.703011344182424,0.620625667064205,0.34727342445389));
#35729=DIRECTION('center_axis',(0.,0.941287071653639,-0.337607240351444));
#35730=DIRECTION('ref_axis',(0.,0.337607240351444,0.941287071653639));
#35731=DIRECTION('',(0.,-0.337607240351444,-0.941287071653639));
#35732=DIRECTION('',(1.,0.,0.));
#35733=DIRECTION('',(-1.,0.,0.));
#35734=DIRECTION('center_axis',(0.707106781186518,0.662164269064559,0.248069507949364));
#35735=DIRECTION('ref_axis',(0.331042401509786,0.,-0.943615879689736));
#35736=DIRECTION('',(0.542846344219036,-0.283533375605797,-0.79052303665713));
#35737=DIRECTION('',(0.,0.350823262553197,-0.936441689829928));
#35738=DIRECTION('',(0.,-0.350823262553197,0.936441689829928));
#35739=DIRECTION('',(0.606604029806706,-0.748327100188909,0.268399147064822));
#35740=DIRECTION('center_axis',(0.707106781186517,0.353553390593289,-0.612372435695821));
#35741=DIRECTION('ref_axis',(-0.65465367070801,0.,-0.755928946018426));
#35742=DIRECTION('',(-0.542846344219037,0.82637971982479,-0.149714412233186));
#35743=DIRECTION('',(0.,0.866025403784439,0.5));
#35744=DIRECTION('',(0.,-0.866025403784439,-0.5));
#35745=DIRECTION('',(-0.60660402980671,-0.14172307038225,-0.782269852636344));
#35746=DIRECTION('center_axis',(0.,0.936441689829928,0.350823262553197));
#35747=DIRECTION('ref_axis',(0.,-0.350823262553197,0.936441689829928));
#35748=DIRECTION('',(0.,0.350823262553197,-0.936441689829928));
#35749=DIRECTION('',(0.,-0.350823262553197,0.936441689829928));
#35750=DIRECTION('',(-0.702246883176787,0.249762834828468,-0.6666842141576));
#35751=DIRECTION('',(-1.,0.,0.));
#35752=DIRECTION('center_axis',(0.,0.5,-0.866025403784439));
#35753=DIRECTION('ref_axis',(0.,0.866025403784439,0.5));
#35754=DIRECTION('',(1.,0.,0.));
#35755=DIRECTION('',(0.,-0.866025403784439,-0.5));
#35756=DIRECTION('center_axis',(0.,-0.178267089180912,-0.983982136481636));
#35757=DIRECTION('ref_axis',(-1.,0.,0.));
#35758=DIRECTION('',(-0.542846344219054,-0.82637971982478,0.149714412233182));
#35759=DIRECTION('',(-1.,0.,0.));
#35760=DIRECTION('',(0.,-0.983982136481636,0.178267089180912));
#35761=DIRECTION('center_axis',(0.617021082541744,-0.774341417050779,0.140286683397983));
#35762=DIRECTION('ref_axis',(0.221703181086956,0.,-0.975114198181897));
#35763=DIRECTION('',(0.701419241812875,0.460329741422837,-0.544157676024363));
#35764=DIRECTION('',(0.,0.178267089180919,0.983982136481635));
#35765=DIRECTION('',(-0.701419241812876,-0.621975132183211,-0.348077551933944));
#35766=DIRECTION('center_axis',(-0.617021082541771,-0.774341417050759,0.140286683397977));
#35767=DIRECTION('ref_axis',(0.221703181086938,0.,0.975114198181901));
#35768=DIRECTION('',(0.,-0.178267089180919,-0.983982136481635));
#35769=DIRECTION('',(0.70141924181285,-0.460329741422853,0.544157676024382));
#35770=DIRECTION('',(-0.701419241812853,0.621975132183231,0.348077551933954));
#35771=DIRECTION('center_axis',(-0.707106781186544,-0.353553390593275,0.612372435695797));
#35772=DIRECTION('ref_axis',(0.654653670707981,0.,0.755928946018452));
#35773=DIRECTION('',(0.,-0.866025403784439,-0.5));
#35774=DIRECTION('',(0.,0.866025403784439,0.5));
#35775=DIRECTION('',(-0.606604029806695,0.748327100188916,-0.268399147064825));
#35776=DIRECTION('center_axis',(-0.707106781186542,-0.545916630320717,-0.449416324513565));
#35777=DIRECTION('ref_axis',(-0.536399063209287,0.,0.843964480880682));
#35778=DIRECTION('',(0.,-0.635570661278947,0.772042702524571));
#35779=DIRECTION('',(0.,0.635570661278947,-0.772042702524571));
#35780=DIRECTION('center_axis',(0.,-0.983982136481635,0.178267089180919));
#35781=DIRECTION('ref_axis',(0.,-0.178267089180919,-0.983982136481635));
#35782=DIRECTION('',(-1.,0.,0.));
#35783=DIRECTION('',(1.,0.,0.));
#35784=DIRECTION('center_axis',(0.707106781186517,-0.545916630320736,-0.449416324513581));
#35785=DIRECTION('ref_axis',(-0.536399063209314,0.,-0.843964480880665));
#35786=DIRECTION('',(0.,-0.635570661278947,0.772042702524571));
#35787=DIRECTION('',(0.,0.635570661278947,-0.772042702524571));
#35788=DIRECTION('center_axis',(0.707106781186519,-0.353553390593288,0.612372435695819));
#35789=DIRECTION('ref_axis',(0.654653670708007,0.,-0.755928946018428));
#35790=DIRECTION('',(0.606604029806723,0.748327100188896,-0.268399147064818));
#35791=DIRECTION('',(0.,-0.866025403784439,-0.5));
#35792=DIRECTION('',(0.,0.866025403784439,0.5));
#35793=DIRECTION('center_axis',(0.,0.33760724035145,0.941287071653637));
#35794=DIRECTION('ref_axis',(1.,0.,0.));
#35795=DIRECTION('',(1.,0.,0.));
#35796=DIRECTION('center_axis',(0.,-0.772042702524571,-0.635570661278947));
#35797=DIRECTION('ref_axis',(0.,0.635570661278947,-0.772042702524571));
#35798=DIRECTION('',(0.,-0.635570661278947,0.772042702524571));
#35799=DIRECTION('center_axis',(1.,0.,0.));
#35800=DIRECTION('ref_axis',(0.,0.,-1.));
#35801=DIRECTION('center_axis',(0.,-0.5,0.866025403784439));
#35802=DIRECTION('ref_axis',(0.,-0.866025403784439,-0.5));
#35803=DIRECTION('center_axis',(0.55328079542486,-0.148495560929736,0.81965201750389));
#35804=DIRECTION('ref_axis',(0.828841319689926,0.,-0.559483750232893));
#35805=DIRECTION('',(0.703011344182424,-0.44457862695077,-0.555089987668116));
#35806=DIRECTION('',(0.,0.983982136481636,0.178267089180912));
#35807=DIRECTION('',(-0.703011344182425,-0.611060441168389,0.363840881691315));
#35808=DIRECTION('center_axis',(0.,-0.178267089180912,0.983982136481636));
#35809=DIRECTION('ref_axis',(1.,0.,0.));
#35810=DIRECTION('',(0.,0.983982136481636,0.178267089180912));
#35811=DIRECTION('',(1.,0.,0.));
#35812=DIRECTION('',(-1.,0.,0.));
#35813=DIRECTION('center_axis',(0.617021082541743,-0.77434141705078,-0.140286683397981));
#35814=DIRECTION('ref_axis',(-0.221703181086953,0.,-0.975114198181898));
#35815=DIRECTION('',(0.701419241812879,0.621975132183207,-0.348077551933945));
#35816=DIRECTION('',(0.,-0.178267089180915,0.983982136481635));
#35817=DIRECTION('',(-0.701419241812875,-0.460329741422837,-0.544157676024363));
#35818=DIRECTION('center_axis',(0.553280795424862,0.784087249886404,0.281225080637571));
#35819=DIRECTION('ref_axis',(0.453113352871861,0.,-0.891452909271836));
#35820=DIRECTION('',(0.703011344182424,-0.620625667064201,0.347273424453897));
#35821=DIRECTION('',(0.,0.337607240351439,-0.941287071653641));
#35822=DIRECTION('',(-0.703011344182424,0.258432717231595,0.66256137875303));
#35823=DIRECTION('center_axis',(0.,0.941287071653641,0.337607240351439));
#35824=DIRECTION('ref_axis',(0.,-0.337607240351439,0.941287071653641));
#35825=DIRECTION('',(0.,0.337607240351439,-0.941287071653641));
#35826=DIRECTION('',(1.,0.,0.));
#35827=DIRECTION('',(-1.,0.,0.));
#35828=DIRECTION('center_axis',(0.707106781186517,0.353553390593289,0.61237243569582));
#35829=DIRECTION('ref_axis',(0.654653670708009,0.,-0.755928946018427));
#35830=DIRECTION('',(0.,0.866025403784438,-0.500000000000001));
#35831=DIRECTION('',(0.,-0.866025403784438,0.500000000000001));
#35832=DIRECTION('center_axis',(-0.617021082541769,-0.77434141705076,-0.140286683397974));
#35833=DIRECTION('ref_axis',(-0.221703181086934,0.,0.975114198181902));
#35834=DIRECTION('',(0.,0.178267089180915,-0.983982136481635));
#35835=DIRECTION('',(0.701419241812854,-0.621975132183229,0.348077551933958));
#35836=DIRECTION('',(-0.70141924181285,0.460329741422853,0.544157676024382));
#35837=DIRECTION('center_axis',(-0.707106781186542,-0.545916630320716,0.449416324513565));
#35838=DIRECTION('ref_axis',(0.536399063209287,0.,0.843964480880682));
#35839=DIRECTION('',(0.,-0.635570661278947,-0.77204270252457));
#35840=DIRECTION('',(0.,0.635570661278947,0.77204270252457));
#35841=DIRECTION('center_axis',(0.617021082541747,0.265678876890073,-0.740742680067404));
#35842=DIRECTION('ref_axis',(-0.768356185646342,0.,-0.640022477713872));
#35843=DIRECTION('',(0.701419241812876,0.241089500389983,0.67073608820188));
#35844=DIRECTION('',(0.,-0.941287071653641,-0.337607240351439));
#35845=DIRECTION('',(-0.701419241812877,0.612431568553495,-0.364607489025876));
#35846=DIRECTION('center_axis',(-0.617021082541771,0.265678876890066,-0.740742680067387));
#35847=DIRECTION('ref_axis',(-0.768356185646323,0.,0.640022477713895));
#35848=DIRECTION('',(0.,0.941287071653641,0.337607240351439));
#35849=DIRECTION('',(0.70141924181285,-0.241089500389991,-0.670736088201903));
#35850=DIRECTION('',(-0.701419241812852,-0.61243156855352,0.364607489025883));
#35851=DIRECTION('center_axis',(-0.707106781186544,-0.353553390593276,-0.612372435695797));
#35852=DIRECTION('ref_axis',(-0.65465367070798,0.,0.755928946018452));
#35853=DIRECTION('',(0.,-0.866025403784438,0.5));
#35854=DIRECTION('',(0.,0.866025403784438,-0.5));
#35855=DIRECTION('center_axis',(-0.707106781186543,0.662164269064536,-0.248069507949356));
#35856=DIRECTION('ref_axis',(-0.331042401509766,0.,0.943615879689743));
#35857=DIRECTION('',(0.,-0.350823262553198,-0.936441689829927));
#35858=DIRECTION('',(0.,0.350823262553198,0.936441689829927));
#35859=DIRECTION('center_axis',(0.,0.337607240351439,-0.941287071653641));
#35860=DIRECTION('ref_axis',(-1.,0.,0.));
#35861=DIRECTION('',(-1.,0.,0.));
#35862=DIRECTION('',(1.,0.,0.));
#35863=DIRECTION('center_axis',(0.707106781186517,0.66216426906456,-0.248069507949365));
#35864=DIRECTION('ref_axis',(-0.331042401509787,0.,-0.943615879689735));
#35865=DIRECTION('',(0.,-0.350823262553198,-0.936441689829927));
#35866=DIRECTION('',(0.,0.350823262553198,0.936441689829927));
#35867=DIRECTION('center_axis',(0.707106781186519,-0.353553390593288,-0.612372435695819));
#35868=DIRECTION('ref_axis',(-0.654653670708007,0.,-0.755928946018429));
#35869=DIRECTION('',(0.,-0.866025403784438,0.5));
#35870=DIRECTION('',(0.,0.866025403784438,-0.5));
#35871=DIRECTION('center_axis',(0.,-0.983982136481635,-0.178267089180915));
#35872=DIRECTION('ref_axis',(0.,0.178267089180915,-0.983982136481635));
#35873=DIRECTION('',(-1.,0.,0.));
#35874=DIRECTION('',(1.,0.,0.));
#35875=DIRECTION('center_axis',(0.707106781186517,-0.545916630320736,0.449416324513581));
#35876=DIRECTION('ref_axis',(0.536399063209314,0.,-0.843964480880665));
#35877=DIRECTION('',(0.,0.635570661278947,0.77204270252457));
#35878=DIRECTION('',(0.,-0.635570661278947,-0.77204270252457));
#35879=DIRECTION('center_axis',(0.,-0.77204270252457,0.635570661278947));
#35880=DIRECTION('ref_axis',(0.,-0.635570661278947,-0.77204270252457));
#35881=DIRECTION('',(0.,0.635570661278947,0.77204270252457));
#35882=DIRECTION('center_axis',(0.,0.500000000000001,0.866025403784438));
#35883=DIRECTION('ref_axis',(0.,-0.866025403784438,0.500000000000001));
#35884=DIRECTION('',(0.,0.866025403784438,-0.500000000000001));
#35885=DIRECTION('center_axis',(1.,0.,0.));
#35886=DIRECTION('ref_axis',(0.,0.,-1.));
#35887=DIRECTION('center_axis',(0.,-0.5,-0.866025403784438));
#35888=DIRECTION('ref_axis',(0.,0.866025403784438,-0.5));
#35889=DIRECTION('',(0.707106781186529,1.96261557335478E-15,-0.707106781186566));
#35890=DIRECTION('center_axis',(0.,0.,-1.));
#35891=DIRECTION('ref_axis',(1.,0.,0.));
#35892=DIRECTION('',(0.,0.,-1.));
#35893=DIRECTION('center_axis',(0.,0.,-1.));
#35894=DIRECTION('ref_axis',(1.,0.,0.));
#35895=DIRECTION('center_axis',(0.,0.,-1.));
#35896=DIRECTION('ref_axis',(1.,0.,0.));
#35897=DIRECTION('center_axis',(0.,0.,1.));
#35898=DIRECTION('ref_axis',(1.,0.,0.));
#35899=DIRECTION('',(-1.,0.,0.));
#35900=DIRECTION('center_axis',(0.,0.,1.));
#35901=DIRECTION('ref_axis',(1.,0.,0.));
#35902=DIRECTION('',(-1.,0.,0.));
#35903=DIRECTION('center_axis',(0.,0.936441689829928,-0.350823262553198));
#35904=DIRECTION('ref_axis',(0.,0.350823262553198,0.936441689829927));
#35905=DIRECTION('',(0.,-0.350823262553198,-0.936441689829927));
#35906=DIRECTION('center_axis',(1.,0.,0.));
#35907=DIRECTION('ref_axis',(0.,0.,-1.));
#35908=DIRECTION('center_axis',(1.,0.,0.));
#35909=DIRECTION('ref_axis',(0.,0.,-1.));
#35910=DIRECTION('center_axis',(0.,-0.164398987305357,0.986393923832144));
#35911=DIRECTION('ref_axis',(0.,-0.986393923832144,-0.164398987305357));
#35912=DIRECTION('',(0.,0.986393923832144,0.164398987305357));
#35913=DIRECTION('center_axis',(1.,0.,0.));
#35914=DIRECTION('ref_axis',(0.,0.,-1.));
#35915=DIRECTION('center_axis',(1.,0.,0.));
#35916=DIRECTION('ref_axis',(0.,-1.83697019872103E-16,-1.));
#35917=DIRECTION('center_axis',(1.,0.,0.));
#35918=DIRECTION('ref_axis',(0.,0.,-1.));
#35919=DIRECTION('',(-1.,0.,0.));
#35920=DIRECTION('',(-1.,0.,0.));
#35921=DIRECTION('center_axis',(1.,0.,0.));
#35922=DIRECTION('ref_axis',(0.,0.,-1.));
#46089=CARTESIAN_POINT('',(0.,0.,0.));
#46090=CARTESIAN_POINT('Origin',(189.823223304703,0.,-7.45612530191356E-16));
#46091=CARTESIAN_POINT('',(190.,-17.6605334048044,15.5034047827497));
#46092=CARTESIAN_POINT('',(189.646446609407,-18.2099328514786,16.170773274433));
#46093=CARTESIAN_POINT('Ctrl Pts',(189.646446609407,-18.2099328514786,16.1707732744329));
#46094=CARTESIAN_POINT('Ctrl Pts',(189.826457221484,-17.9303333695711,15.8311371760613));
#46095=CARTESIAN_POINT('Ctrl Pts',(190.,-17.6605334048044,15.5034047827497));
#46096=CARTESIAN_POINT('',(189.646446609407,-24.3535533905933,-2.98245012076542E-15));
#46097=CARTESIAN_POINT('Origin',(189.646446609407,0.,-1.49122506038271E-15));
#46098=CARTESIAN_POINT('',(189.646446609407,-18.2099328514786,-16.170773274433));
#46099=CARTESIAN_POINT('Origin',(189.646446609407,0.,-1.49122506038271E-15));
#46100=CARTESIAN_POINT('',(190.,-17.6605334048044,-15.5034047827497));
#46101=CARTESIAN_POINT('Ctrl Pts',(190.,-17.6605334048045,-15.5034047827498));
#46102=CARTESIAN_POINT('Ctrl Pts',(189.826457222012,-17.9303333687502,-15.831137175064));
#46103=CARTESIAN_POINT('Ctrl Pts',(189.646446609407,-18.2099328514788,-16.1707732744332));
#46104=CARTESIAN_POINT('Origin',(190.,0.,0.));
#46105=CARTESIAN_POINT('Origin',(189.5,0.,0.));
#46106=CARTESIAN_POINT('',(190.,-17.9824248820024,-15.8944139672761));
#46107=CARTESIAN_POINT('Ctrl Pts',(189.646446609407,-18.2099328514786,-16.170773274433));
#46108=CARTESIAN_POINT('Ctrl Pts',(189.824548278075,-18.0953471159447,-16.0315832735063));
#46109=CARTESIAN_POINT('Ctrl Pts',(190.,-17.9824248820024,-15.8944139672761));
#46110=CARTESIAN_POINT('',(189.353553390593,-24.6464466094067,-3.01831919505661E-15));
#46111=CARTESIAN_POINT('',(189.5,-24.5,-3.00038465791102E-15));
#46112=CARTESIAN_POINT('',(189.353553390593,24.6464466094067,-3.01831919505661E-15));
#46113=CARTESIAN_POINT('Origin',(189.353553390593,0.,-1.5091595975283E-15));
#46114=CARTESIAN_POINT('Origin',(189.353553390593,0.,-1.5091595975283E-15));
#46115=CARTESIAN_POINT('',(190.,-17.9824248820024,15.8944139672761));
#46116=CARTESIAN_POINT('Ctrl Pts',(190.,-17.9824248820024,15.8944139672761));
#46117=CARTESIAN_POINT('Ctrl Pts',(189.824548278098,-18.0953471159299,16.0315832734883));
#46118=CARTESIAN_POINT('Ctrl Pts',(189.646446609407,-18.2099328514786,16.170773274433));
#46119=CARTESIAN_POINT('',(190.5,-17.6605334048044,15.5034047827497));
#46120=CARTESIAN_POINT('Ctrl Pts',(190.,-17.9824248820024,15.8944139672761));
#46121=CARTESIAN_POINT('Ctrl Pts',(190.252700024269,-17.8197849777336,15.6968514319361));
#46122=CARTESIAN_POINT('Ctrl Pts',(190.5,-17.6605334048044,15.5034047827497));
#46123=CARTESIAN_POINT('',(190.,-17.6436771757118,16.2696237116679));
#46124=CARTESIAN_POINT('Ctrl Pts',(190.499999999993,-17.6605334048042,15.5034047827607));
#46125=CARTESIAN_POINT('Ctrl Pts',(190.253091651642,-17.65449217735,15.8845492841333));
#46126=CARTESIAN_POINT('Ctrl Pts',(190.,-17.6436771757118,16.2696237116679));
#46127=CARTESIAN_POINT('',(190.,-4.77375383292611,23.5204437530975));
#46128=CARTESIAN_POINT('Origin',(190.,0.,0.));
#46129=CARTESIAN_POINT('',(189.646446609407,-4.89933402875813,23.8556510878058));
#46130=CARTESIAN_POINT('Ctrl Pts',(189.646446609407,-4.89933402875813,23.8556510878058));
#46131=CARTESIAN_POINT('Ctrl Pts',(189.82454827809,-4.83608481976441,23.6868219294443));
#46132=CARTESIAN_POINT('Ctrl Pts',(190.,-4.77375383292611,23.5204437530975));
#46133=CARTESIAN_POINT('',(189.646446609407,23.1092668802368,7.68487781337279));
#46134=CARTESIAN_POINT('Origin',(189.646446609407,0.,-1.49122506038271E-15));
#46135=CARTESIAN_POINT('',(190.,22.7561787149285,7.62602978582142));
#46136=CARTESIAN_POINT('Ctrl Pts',(190.,22.7561787149285,7.62602978582142));
#46137=CARTESIAN_POINT('Ctrl Pts',(189.824548278069,22.9314319357209,7.65523865595349));
#46138=CARTESIAN_POINT('Ctrl Pts',(189.646446609407,23.1092668802368,7.68487781337279));
#46139=CARTESIAN_POINT('',(190.5,22.2566090894166,7.54276818156944));
#46140=CARTESIAN_POINT('Ctrl Pts',(190.,22.7561787149285,7.62602978582142));
#46141=CARTESIAN_POINT('Ctrl Pts',(190.252700024268,22.5037645883542,7.58396076472571));
#46142=CARTESIAN_POINT('Ctrl Pts',(190.5,22.2566090894167,7.54276818156944));
#46143=CARTESIAN_POINT('',(190.,22.911746032174,7.14506079450414));
#46144=CARTESIAN_POINT('Ctrl Pts',(190.499999999993,22.2566090894261,7.5427681815638));
#46145=CARTESIAN_POINT('Ctrl Pts',(190.253091651642,22.5836692964003,7.34696407443207));
#46146=CARTESIAN_POINT('Ctrl Pts',(190.,22.911746032174,7.14506079450414));
#46147=CARTESIAN_POINT('',(190.,22.911746032174,-7.14506079450414));
#46148=CARTESIAN_POINT('Origin',(190.,0.,0.));
#46149=CARTESIAN_POINT('',(190.5,22.2566090894166,-7.54276818156944));
#46150=CARTESIAN_POINT('Ctrl Pts',(190.,22.911746032174,-7.14506079450415));
#46151=CARTESIAN_POINT('Ctrl Pts',(190.253091651653,22.5836692963867,-7.34696407444047));
#46152=CARTESIAN_POINT('Ctrl Pts',(190.500000000013,22.2566090893989,-7.54276818158009));
#46153=CARTESIAN_POINT('',(190.,22.7561787149285,-7.62602978582142));
#46154=CARTESIAN_POINT('Ctrl Pts',(190.5,22.2566090894167,-7.54276818156944));
#46155=CARTESIAN_POINT('Ctrl Pts',(190.252700024268,22.5037645883541,-7.58396076472568));
#46156=CARTESIAN_POINT('Ctrl Pts',(190.,22.7561787149285,-7.62602978582142));
#46157=CARTESIAN_POINT('',(189.646446609407,23.1092668802368,-7.6848778133728));
#46158=CARTESIAN_POINT('Ctrl Pts',(189.646446609407,23.1092668802368,-7.6848778133728));
#46159=CARTESIAN_POINT('Ctrl Pts',(189.824548278069,22.9314319357209,-7.65523865595349));
#46160=CARTESIAN_POINT('Ctrl Pts',(190.,22.7561787149285,-7.62602978582142));
#46161=CARTESIAN_POINT('',(189.646446609407,-4.89933402875815,-23.8556510878058));
#46162=CARTESIAN_POINT('Origin',(189.646446609407,0.,-1.49122506038271E-15));
#46163=CARTESIAN_POINT('',(190.,-4.77375383292613,-23.5204437530975));
#46164=CARTESIAN_POINT('Ctrl Pts',(190.,-4.77375383292613,-23.5204437530975));
#46165=CARTESIAN_POINT('Ctrl Pts',(189.824548278103,-4.83608481975967,-23.6868219294316));
#46166=CARTESIAN_POINT('Ctrl Pts',(189.646446609407,-4.89933402875815,-23.8556510878058));
#46167=CARTESIAN_POINT('',(190.5,-4.59607568461225,-23.0461729643192));
#46168=CARTESIAN_POINT('Ctrl Pts',(190.,-4.77375383292613,-23.5204437530975));
#46169=CARTESIAN_POINT('Ctrl Pts',(190.252700024269,-4.6839796106199,-23.2808121966615));
#46170=CARTESIAN_POINT('Ctrl Pts',(190.5,-4.59607568461225,-23.0461729643192));
#46171=CARTESIAN_POINT('',(190.,-5.26806885646218,-23.414684506172));
#46172=CARTESIAN_POINT('Ctrl Pts',(190.499999999993,-4.59607568462184,-23.0461729643245));
#46173=CARTESIAN_POINT('Ctrl Pts',(190.253091651642,-4.92917711905038,-23.2315133585654));
#46174=CARTESIAN_POINT('Ctrl Pts',(190.,-5.26806885646218,-23.414684506172));
#46175=CARTESIAN_POINT('',(190.,-17.6436771757118,-16.2696237116679));
#46176=CARTESIAN_POINT('Origin',(190.,0.,0.));
#46177=CARTESIAN_POINT('',(190.5,-17.6605334048044,-15.5034047827497));
#46178=CARTESIAN_POINT('Ctrl Pts',(190.,-17.6436771757118,-16.2696237116679));
#46179=CARTESIAN_POINT('Ctrl Pts',(190.253091651653,-17.6544921773504,-15.8845492841173));
#46180=CARTESIAN_POINT('Ctrl Pts',(190.500000000013,-17.6605334048048,-15.503404782729));
#46181=CARTESIAN_POINT('Ctrl Pts',(190.5,-17.6605334048044,-15.5034047827497));
#46182=CARTESIAN_POINT('Ctrl Pts',(190.252700024271,-17.819784977732,-15.696851431934));
#46183=CARTESIAN_POINT('Ctrl Pts',(190.,-17.9824248820024,-15.8944139672761));
#46184=CARTESIAN_POINT('Origin',(160.176776695297,0.,-7.45612530191356E-16));
#46185=CARTESIAN_POINT('',(160.353553390593,24.3535533905933,-2.98245012076542E-15));
#46186=CARTESIAN_POINT('',(160.353553390593,-24.3535533905933,-2.98245012076542E-15));
#46187=CARTESIAN_POINT('Origin',(160.353553390593,0.,-1.49122506038271E-15));
#46188=CARTESIAN_POINT('Origin',(160.353553390593,0.,-1.49122506038271E-15));
#46189=CARTESIAN_POINT('',(160.,23.5,2.87791997799628E-15));
#46190=CARTESIAN_POINT('',(160.176776695297,23.9267766952966,2.93018504938085E-15));
#46191=CARTESIAN_POINT('Origin',(160.,0.,0.));
#46192=CARTESIAN_POINT('Origin',(160.5,0.,0.));
#46193=CARTESIAN_POINT('',(160.646446609407,24.6464466094067,3.01831919505661E-15));
#46194=CARTESIAN_POINT('',(160.646446609407,-24.6464466094067,-3.01831919505661E-15));
#46195=CARTESIAN_POINT('Origin',(160.646446609407,0.,-1.5091595975283E-15));
#46196=CARTESIAN_POINT('Origin',(160.646446609407,0.,-1.5091595975283E-15));
#46197=CARTESIAN_POINT('',(160.5,-24.5,-3.00038465791102E-15));
#46198=CARTESIAN_POINT('Origin',(160.,24.,0.));
#46199=CARTESIAN_POINT('',(160.,6.12323399573677E-16,10.));
#46200=CARTESIAN_POINT('Origin',(160.,0.,0.));
#46201=CARTESIAN_POINT('Origin',(189.823223304703,0.,-7.45612530191356E-16));
#46202=CARTESIAN_POINT('',(190.,-4.59607568461223,23.0461729643192));
#46203=CARTESIAN_POINT('Ctrl Pts',(190.,-4.5960756846122,23.0461729643191));
#46204=CARTESIAN_POINT('Ctrl Pts',(189.826457221778,-4.74500028022709,23.4436927837287));
#46205=CARTESIAN_POINT('Ctrl Pts',(189.646446609407,-4.8993340287581,23.8556510878057));
#46206=CARTESIAN_POINT('',(190.,22.2566090894166,7.54276818156944));
#46207=CARTESIAN_POINT('Origin',(190.,0.,0.));
#46208=CARTESIAN_POINT('Ctrl Pts',(189.646446609407,23.1092668802367,7.68487781337279));
#46209=CARTESIAN_POINT('Ctrl Pts',(189.82645722158,22.6753336498196,7.61255560830327));
#46210=CARTESIAN_POINT('Ctrl Pts',(190.,22.2566090894167,7.54276818156945));
#46211=CARTESIAN_POINT('Origin',(189.823223304703,0.,-7.45612530191356E-16));
#46212=CARTESIAN_POINT('',(190.,-4.59607568461224,-23.0461729643192));
#46213=CARTESIAN_POINT('Ctrl Pts',(189.646446609407,-4.89933402875824,-23.855651087806));
#46214=CARTESIAN_POINT('Ctrl Pts',(189.826457222167,-4.74500027989357,-23.4436927828384));
#46215=CARTESIAN_POINT('Ctrl Pts',(190.,-4.5960756846123,-23.0461729643193));
#46216=CARTESIAN_POINT('',(190.,22.2566090894166,-7.54276818156944));
#46217=CARTESIAN_POINT('Ctrl Pts',(190.,22.2566090894165,-7.54276818156942));
#46218=CARTESIAN_POINT('Ctrl Pts',(189.826457222193,22.6753336483417,-7.61255560805694));
#46219=CARTESIAN_POINT('Ctrl Pts',(189.646446609407,23.1092668802368,-7.68487781337279));
#46220=CARTESIAN_POINT('Origin',(190.,0.,0.));
#46221=CARTESIAN_POINT('Origin',(195.5,13.4931969619161,-6.08219949365268));
#46222=CARTESIAN_POINT('',(195.5,13.,-5.5));
#46223=CARTESIAN_POINT('',(196.,13.5,-5.57643645580848));
#46224=CARTESIAN_POINT('',(195.5,13.,-5.5));
#46225=CARTESIAN_POINT('',(195.5,13.4931969619161,-6.08219949365268));
#46226=CARTESIAN_POINT('',(195.5,13.4931969619161,-6.08219949365268));
#46227=CARTESIAN_POINT('',(196.,13.5,-5.57643645580848));
#46228=CARTESIAN_POINT('Origin',(190.,13.246598480958,-5.79109974682634));
#46229=CARTESIAN_POINT('',(190.,13.,-5.5));
#46230=CARTESIAN_POINT('',(190.,13.4931969619161,-6.08219949365268));
#46231=CARTESIAN_POINT('',(190.,11.1403068356888,-3.3047058229942));
#46232=CARTESIAN_POINT('',(190.,13.4931969619161,-6.08219949365268));
#46233=CARTESIAN_POINT('',(190.,13.,-5.5));
#46234=CARTESIAN_POINT('Origin',(195.5,25.,-7.5));
#46235=CARTESIAN_POINT('',(195.5,24.5068030380839,-7.91780050634732));
#46236=CARTESIAN_POINT('',(196.,24.5,-7.40976978914182));
#46237=CARTESIAN_POINT('',(195.5,24.5068030380839,-7.91780050634732));
#46238=CARTESIAN_POINT('',(195.5,25.,-7.5));
#46239=CARTESIAN_POINT('',(195.5,25.,-7.5));
#46240=CARTESIAN_POINT('',(196.,24.5,-7.40976978914182));
#46241=CARTESIAN_POINT('Origin',(195.5,13.,5.5));
#46242=CARTESIAN_POINT('',(195.5,13.4931969619161,6.08219949365268));
#46243=CARTESIAN_POINT('',(196.,13.5,5.57643645580848));
#46244=CARTESIAN_POINT('',(195.5,13.4931969619161,6.08219949365268));
#46245=CARTESIAN_POINT('',(195.5,13.,5.5));
#46246=CARTESIAN_POINT('',(195.5,13.,5.5));
#46247=CARTESIAN_POINT('',(196.,13.5,5.57643645580848));
#46248=CARTESIAN_POINT('Origin',(190.,13.246598480958,5.79109974682634));
#46249=CARTESIAN_POINT('',(190.,13.4931969619161,6.08219949365268));
#46250=CARTESIAN_POINT('',(190.,13.,5.5));
#46251=CARTESIAN_POINT('',(190.,11.1403068356888,3.30470582299419));
#46252=CARTESIAN_POINT('',(190.,13.,5.5));
#46253=CARTESIAN_POINT('',(190.,13.4931969619161,6.08219949365268));
#46254=CARTESIAN_POINT('Origin',(195.75,13.25,3.));
#46255=CARTESIAN_POINT('',(196.,13.5,3.));
#46256=CARTESIAN_POINT('',(195.5,13.,3.));
#46257=CARTESIAN_POINT('Origin',(190.,24.5,-7.40976978914182));
#46258=CARTESIAN_POINT('',(190.5,24.5068030380839,-7.91780050634732));
#46259=CARTESIAN_POINT('',(190.5,25.,-7.5));
#46260=CARTESIAN_POINT('',(190.5,24.5068030380839,-7.91780050634732));
#46261=CARTESIAN_POINT('',(190.,24.5,-7.40976978914182));
#46262=CARTESIAN_POINT('',(190.,24.5,-7.40976978914182));
#46263=CARTESIAN_POINT('',(190.5,25.,-7.5));
#46264=CARTESIAN_POINT('Origin',(190.25,15.4735321792588,-6.15880692444737));
#46265=CARTESIAN_POINT('',(190.,15.5146319260851,-5.91220844348933));
#46266=CARTESIAN_POINT('',(190.5,15.4324324324324,-6.40540540540541));
#46267=CARTESIAN_POINT('Origin',(195.5,24.5068030380839,7.91780050634732));
#46268=CARTESIAN_POINT('',(195.5,25.,7.5));
#46269=CARTESIAN_POINT('',(196.,24.5,7.40976978914182));
#46270=CARTESIAN_POINT('',(195.5,25.,7.5));
#46271=CARTESIAN_POINT('',(195.5,24.5068030380839,7.91780050634732));
#46272=CARTESIAN_POINT('',(195.5,24.5068030380839,7.91780050634732));
#46273=CARTESIAN_POINT('',(196.,24.5,7.40976978914182));
#46274=CARTESIAN_POINT('Origin',(190.,24.5,7.40976978914181));
#46275=CARTESIAN_POINT('',(190.5,25.,7.5));
#46276=CARTESIAN_POINT('',(190.5,24.5068030380839,7.91780050634732));
#46277=CARTESIAN_POINT('',(190.5,25.,7.5));
#46278=CARTESIAN_POINT('',(190.,24.5,7.40976978914182));
#46279=CARTESIAN_POINT('',(190.,24.5,7.40976978914181));
#46280=CARTESIAN_POINT('',(190.5,24.5068030380839,7.91780050634732));
#46281=CARTESIAN_POINT('Origin',(190.25,24.75,-4.));
#46282=CARTESIAN_POINT('',(190.5,25.,-4.));
#46283=CARTESIAN_POINT('',(190.,24.5,-4.));
#46284=CARTESIAN_POINT('Origin',(190.25,21.4735321792588,7.15880692444737));
#46285=CARTESIAN_POINT('',(190.5,21.4324324324324,7.40540540540541));
#46286=CARTESIAN_POINT('',(190.,21.5146319260851,6.91220844348933));
#46287=CARTESIAN_POINT('Origin',(190.,24.753401519042,7.70890025317366));
#46288=CARTESIAN_POINT('',(190.,25.,7.5));
#46289=CARTESIAN_POINT('',(190.,24.5068030380839,7.91780050634732));
#46290=CARTESIAN_POINT('Origin',(195.75,21.4735321792588,7.15880692444737));
#46291=CARTESIAN_POINT('',(196.,21.5146319260851,6.91220844348934));
#46292=CARTESIAN_POINT('',(195.5,21.4324324324324,7.40540540540541));
#46293=CARTESIAN_POINT('Origin',(195.75,24.75,-4.));
#46294=CARTESIAN_POINT('',(196.,24.5,-4.));
#46295=CARTESIAN_POINT('',(195.5,25.,-4.));
#46296=CARTESIAN_POINT('Origin',(190.,24.753401519042,-7.70890025317366));
#46297=CARTESIAN_POINT('',(190.,24.5068030380839,-7.91780050634732));
#46298=CARTESIAN_POINT('',(190.,25.,-7.5));
#46299=CARTESIAN_POINT('Origin',(195.75,15.4735321792588,-6.15880692444737));
#46300=CARTESIAN_POINT('',(196.,15.5146319260851,-5.91220844348933));
#46301=CARTESIAN_POINT('',(195.5,15.4324324324324,-6.40540540540541));
#46302=CARTESIAN_POINT('Origin',(190.,13.,-6.));
#46303=CARTESIAN_POINT('',(190.,11.0540540540541,-5.67567567567568));
#46304=CARTESIAN_POINT('Origin',(190.,13.,6.));
#46305=CARTESIAN_POINT('',(190.,13.,3.));
#46306=CARTESIAN_POINT('Origin',(196.,19.,0.));
#46307=CARTESIAN_POINT('Origin',(190.,25.,-8.));
#46308=CARTESIAN_POINT('Origin',(161.073223304703,0.,-7.54579798764152E-16));
#46309=CARTESIAN_POINT('',(161.5,25.,-3.06161699786838E-15));
#46310=CARTESIAN_POINT('',(161.5,-25.,-3.06161699786838E-15));
#46311=CARTESIAN_POINT('Origin',(161.5,0.,0.));
#46312=CARTESIAN_POINT('Origin',(161.5,0.,0.));
#46313=CARTESIAN_POINT('',(161.073223304703,24.8232233047034,3.0399680964625E-15));
#46314=CARTESIAN_POINT('Origin',(175.,0.,0.));
#46315=CARTESIAN_POINT('',(188.5,25.,3.06161699786838E-15));
#46316=CARTESIAN_POINT('',(188.5,-25.,-3.06161699786838E-15));
#46317=CARTESIAN_POINT('Origin',(188.5,0.,0.));
#46318=CARTESIAN_POINT('Origin',(188.5,0.,0.));
#46319=CARTESIAN_POINT('',(175.,-25.,-3.06161699786838E-15));
#46320=CARTESIAN_POINT('',(168.1,-5.27355936696949E-15,25.));
#46321=CARTESIAN_POINT('Ctrl Pts',(168.1,-5.27355936696949E-15,25.));
#46322=CARTESIAN_POINT('Ctrl Pts',(168.1,-0.55163791047639,25.));
#46323=CARTESIAN_POINT('Ctrl Pts',(168.267431880558,-1.33721306717284,24.9721836184323));
#46324=CARTESIAN_POINT('Ctrl Pts',(168.855166000548,-2.3552917259163,24.8917927252736));
#46325=CARTESIAN_POINT('Ctrl Pts',(169.472757569434,-3.03716583184694,24.8179083643489));
#46326=CARTESIAN_POINT('Ctrl Pts',(170.143631676592,-3.44706604659973,24.7613408689562));
#46327=CARTESIAN_POINT('Ctrl Pts',(170.985290745162,-3.79588962505944,24.7105170302552));
#46328=CARTESIAN_POINT('Ctrl Pts',(171.508328520708,-3.89399419357905,24.6944572637537));
#46329=CARTESIAN_POINT('Ctrl Pts',(172.245040749362,-3.89326696112091,24.6947095740839));
#46330=CARTESIAN_POINT('Ctrl Pts',(172.752744962911,-3.8461850836113,24.7021619625942));
#46331=CARTESIAN_POINT('Ctrl Pts',(173.254085442162,-3.6963447003694,24.7252038218524));
#46332=CARTESIAN_POINT('Ctrl Pts',(174.336500109069,-3.24570229252571,24.790351880959));
#46333=CARTESIAN_POINT('Ctrl Pts',(175.349399920632,-2.33707446060684,24.9151419492839));
#46334=CARTESIAN_POINT('Ctrl Pts',(175.870653276153,-0.779198836510287,
24.995496028175));
#46335=CARTESIAN_POINT('Ctrl Pts',(175.909743056997,-0.0151962230191145,
25.0015962526685));
#46336=CARTESIAN_POINT('Ctrl Pts',(175.882356256358,0.418804816251774,24.9973027627956));
#46337=CARTESIAN_POINT('Ctrl Pts',(175.782240123002,1.08365275900373,24.9819016623594));
#46338=CARTESIAN_POINT('Ctrl Pts',(175.489157477974,1.84426230866362,24.937097682422));
#46339=CARTESIAN_POINT('Ctrl Pts',(174.958007340146,2.56739388230451,24.8693513631287));
#46340=CARTESIAN_POINT('Ctrl Pts',(174.346236594584,3.16619529082572,24.8015572991169));
#46341=CARTESIAN_POINT('Ctrl Pts',(173.337625674135,3.74893731769736,24.7187859134922));
#46342=CARTESIAN_POINT('Ctrl Pts',(172.429820467936,3.89494883801314,24.6944680938334));
#46343=CARTESIAN_POINT('Ctrl Pts',(171.509209330769,3.8953602168609,24.694365273583));
#46344=CARTESIAN_POINT('Ctrl Pts',(170.463418858553,3.69742950735511,24.727449381457));
#46345=CARTESIAN_POINT('Ctrl Pts',(169.587124183002,3.10037920374213,24.8094680053816));
#46346=CARTESIAN_POINT('Ctrl Pts',(168.895370153156,2.41044277844561,24.886002008101));
#46347=CARTESIAN_POINT('Ctrl Pts',(168.595968837042,1.9730248402679,24.926626355682));
#46348=CARTESIAN_POINT('Ctrl Pts',(168.197927739773,1.01300388320702,24.9841804475316));
#46349=CARTESIAN_POINT('Ctrl Pts',(168.1,0.490342890750044,25.));
#46350=CARTESIAN_POINT('Ctrl Pts',(168.1,4.71844785465692E-15,25.));
#46351=CARTESIAN_POINT('Origin',(188.926776695297,0.,-7.54579798764152E-16));
#46352=CARTESIAN_POINT('',(188.926776695297,24.8232233047034,3.0399680964625E-15));
#46353=CARTESIAN_POINT('Origin',(195.5,-1.47925920856996,14.7265510941127));
#46354=CARTESIAN_POINT('',(195.5,-1.73686027918559,14.0083302491977));
#46355=CARTESIAN_POINT('',(196.,-1.92066436668019,14.4795611789942));
#46356=CARTESIAN_POINT('',(195.5,-1.73686027918559,14.0083302491977));
#46357=CARTESIAN_POINT('',(195.5,-1.47925920856996,14.7265510941127));
#46358=CARTESIAN_POINT('',(195.5,-1.47925920856996,14.7265510941127));
#46359=CARTESIAN_POINT('',(196.,-1.92066436668019,14.4795611789942));
#46360=CARTESIAN_POINT('Origin',(190.,-1.60805974387777,14.3674406716552));
#46361=CARTESIAN_POINT('',(190.,-1.73686027918559,14.0083302491977));
#46362=CARTESIAN_POINT('',(190.,-1.47925920856996,14.7265510941127));
#46363=CARTESIAN_POINT('',(190.,-3.22940520398334,9.84694662451038));
#46364=CARTESIAN_POINT('',(190.,-1.47925920856996,14.7265510941127));
#46365=CARTESIAN_POINT('',(190.,-1.73686027918559,14.0083302491977));
#46366=CARTESIAN_POINT('Origin',(195.75,-2.53850810591948,16.8413619022243));
#46367=CARTESIAN_POINT('',(195.746598480958,-5.7005973050323,25.2915246721535));
#46368=CARTESIAN_POINT('',(196.,-5.83295112640872,24.9225072872897));
#46369=CARTESIAN_POINT('',(198.006448117623,-6.88093646116468,22.0006059505128));
#46370=CARTESIAN_POINT('',(196.,-2.77261852837696,16.753656086586));
#46371=CARTESIAN_POINT('',(195.5,-5.39638513844789,25.182414249696));
#46372=CARTESIAN_POINT('',(195.5,-2.304397683462,16.9290677178626));
#46373=CARTESIAN_POINT('',(193.284350279285,-2.66308524417351,24.2020737540619));
#46374=CARTESIAN_POINT('Origin',(195.75,-9.43958256229942,9.84983660014381));
#46375=CARTESIAN_POINT('',(195.746598480958,-11.6385387370803,8.57634092482885));
#46376=CARTESIAN_POINT('',(195.5,-11.2631397208144,8.50833024919771));
#46377=CARTESIAN_POINT('',(194.458916574697,-9.67828935113165,8.22120444506385));
#46378=CARTESIAN_POINT('',(195.5,-9.31458256229942,9.63333024919771));
#46379=CARTESIAN_POINT('',(196.,-11.5793356333198,8.90312472318568));
#46380=CARTESIAN_POINT('',(196.,-9.56458256229942,10.0663429510899));
#46381=CARTESIAN_POINT('',(197.517960591876,-11.2246890678024,10.8606699259324));
#46382=CARTESIAN_POINT('Origin',(190.,-1.30384757729337,14.2583302491977));
#46383=CARTESIAN_POINT('',(190.,1.73388677209908,6.14979985501346));
#46384=CARTESIAN_POINT('',(190.,-5.39396555337319,25.1759557260521));
#46385=CARTESIAN_POINT('',(190.,-1.30384757729337,14.2583302491977));
#46386=CARTESIAN_POINT('',(190.006803038084,-5.39638513844789,25.182414249696));
#46387=CARTESIAN_POINT('',(187.037671232877,-4.34037649759326,22.3636430287683));
#46388=CARTESIAN_POINT('',(190.,-5.39638513844789,25.182414249696));
#46389=CARTESIAN_POINT('Origin',(190.,-11.6961524227066,8.25833024919771));
#46390=CARTESIAN_POINT('',(190.,-11.2631397208144,8.50833024919771));
#46391=CARTESIAN_POINT('',(190.,-11.2631397208144,8.50833024919771));
#46392=CARTESIAN_POINT('',(190.,-5.34807621135331,11.9233937586588));
#46393=CARTESIAN_POINT('Origin',(190.,-11.6385387370803,8.57634092482885));
#46394=CARTESIAN_POINT('',(195.5,-12.0139377533461,8.64435160045999));
#46395=CARTESIAN_POINT('',(195.993196961916,-11.2631397208144,8.50833024919771));
#46396=CARTESIAN_POINT('',(190.,-12.0139377533461,8.64435160045999));
#46397=CARTESIAN_POINT('',(190.,-12.0139377533461,8.64435160045999));
#46398=CARTESIAN_POINT('',(190.,-0.410901631705506,6.54224080151618));
#46399=CARTESIAN_POINT('Origin',(195.5,-19.110417899636,17.2646137433487));
#46400=CARTESIAN_POINT('',(195.5,-18.9951905283833,17.900635094611));
#46401=CARTESIAN_POINT('',(196.,-18.6670488735913,17.5127374981478));
#46402=CARTESIAN_POINT('',(195.5,-18.9951905283833,17.900635094611));
#46403=CARTESIAN_POINT('',(195.5,-19.110417899636,17.2646137433487));
#46404=CARTESIAN_POINT('',(195.5,-19.110417899636,17.2646137433487));
#46405=CARTESIAN_POINT('',(196.,-18.6670488735913,17.5127374981478));
#46406=CARTESIAN_POINT('Origin',(190.,-18.6670488735913,17.5127374981478));
#46407=CARTESIAN_POINT('',(190.5,-18.9951905283833,17.900635094611));
#46408=CARTESIAN_POINT('',(190.5,-19.110417899636,17.2646137433487));
#46409=CARTESIAN_POINT('',(190.5,-18.9951905283833,17.900635094611));
#46410=CARTESIAN_POINT('',(190.,-18.6670488735913,17.5127374981478));
#46411=CARTESIAN_POINT('',(190.,-18.6670488735913,17.5127374981478));
#46412=CARTESIAN_POINT('',(190.5,-19.110417899636,17.2646137433487));
#46413=CARTESIAN_POINT('Origin',(190.25,-9.12740473580835,23.3091287436649));
#46414=CARTESIAN_POINT('',(190.,-9.00240473580835,23.0926223927187));
#46415=CARTESIAN_POINT('',(190.5,-6.0048094716167,25.400635094611));
#46416=CARTESIAN_POINT('',(190.5,-9.25240473580835,23.525635094611));
#46417=CARTESIAN_POINT('',(190.5,-6.0048094716167,25.400635094611));
#46418=CARTESIAN_POINT('Origin',(190.25,-17.2340621790159,15.3787074004835));
#46419=CARTESIAN_POINT('',(190.5,-17.4270728546471,15.2198147351638));
#46420=CARTESIAN_POINT('',(190.,-17.0410515033848,15.5376000658033));
#46421=CARTESIAN_POINT('Origin',(190.,-19.0528042140097,17.5826244189798));
#46422=CARTESIAN_POINT('',(190.,-18.9951905283833,17.900635094611));
#46423=CARTESIAN_POINT('',(190.,-19.110417899636,17.2646137433487));
#46424=CARTESIAN_POINT('Origin',(195.75,-17.2340621790159,15.3787074004835));
#46425=CARTESIAN_POINT('',(196.,-17.0410515033848,15.5376000658033));
#46426=CARTESIAN_POINT('',(195.5,-17.4270728546471,15.2198147351638));
#46427=CARTESIAN_POINT('Origin',(195.75,-9.12740473580835,23.3091287436649));
#46428=CARTESIAN_POINT('',(195.5,-6.0048094716167,25.400635094611));
#46429=CARTESIAN_POINT('',(195.5,-6.0048094716167,25.400635094611));
#46430=CARTESIAN_POINT('',(195.5,-9.25240473580835,23.525635094611));
#46431=CARTESIAN_POINT('',(196.,-9.00240473580835,23.0926223927187));
#46432=CARTESIAN_POINT('Origin',(190.,-5.7005973050323,25.2915246721535));
#46433=CARTESIAN_POINT('',(190.,-6.0048094716167,25.400635094611));
#46434=CARTESIAN_POINT('Origin',(190.,-19.4282032302755,17.650635094611));
#46435=CARTESIAN_POINT('',(190.,-9.15396622993757,5.17027660204442));
#46436=CARTESIAN_POINT('Origin',(190.,-10.3660254037844,16.9544826719043));
#46437=CARTESIAN_POINT('Origin',(190.,-5.57179676972449,25.650635094611));
#46438=CARTESIAN_POINT('Origin',(195.5,-12.0139377533461,-8.64435160045998));
#46439=CARTESIAN_POINT('',(195.5,-11.2631397208144,-8.50833024919769));
#46440=CARTESIAN_POINT('',(196.,-11.5793356333198,-8.90312472318567));
#46441=CARTESIAN_POINT('',(195.5,-11.2631397208144,-8.50833024919769));
#46442=CARTESIAN_POINT('',(195.5,-12.0139377533461,-8.64435160045998));
#46443=CARTESIAN_POINT('',(195.5,-12.0139377533461,-8.64435160045998));
#46444=CARTESIAN_POINT('',(196.,-11.5793356333198,-8.90312472318567));
#46445=CARTESIAN_POINT('Origin',(190.,-11.6385387370803,-8.57634092482884));
#46446=CARTESIAN_POINT('',(190.,-11.2631397208144,-8.5083302491977));
#46447=CARTESIAN_POINT('',(190.,-12.0139377533461,-8.64435160045998));
#46448=CARTESIAN_POINT('',(190.,-0.410901631705511,-6.54224080151617));
#46449=CARTESIAN_POINT('',(190.,-12.0139377533461,-8.64435160045998));
#46450=CARTESIAN_POINT('',(190.,-11.2631397208144,-8.50833024919769));
#46451=CARTESIAN_POINT('Origin',(195.5,-18.9951905283833,-17.900635094611));
#46452=CARTESIAN_POINT('',(195.5,-19.110417899636,-17.2646137433487));
#46453=CARTESIAN_POINT('',(196.,-18.6670488735913,-17.5127374981478));
#46454=CARTESIAN_POINT('',(195.5,-19.110417899636,-17.2646137433487));
#46455=CARTESIAN_POINT('',(195.5,-18.9951905283833,-17.900635094611));
#46456=CARTESIAN_POINT('',(195.5,-18.9951905283833,-17.900635094611));
#46457=CARTESIAN_POINT('',(196.,-18.6670488735913,-17.5127374981478));
#46458=CARTESIAN_POINT('Origin',(195.5,-1.73686027918559,-14.0083302491977));
#46459=CARTESIAN_POINT('',(195.5,-1.47925920856997,-14.7265510941127));
#46460=CARTESIAN_POINT('',(196.,-1.9206643666802,-14.4795611789942));
#46461=CARTESIAN_POINT('',(195.5,-1.47925920856997,-14.7265510941127));
#46462=CARTESIAN_POINT('',(195.5,-1.73686027918559,-14.0083302491977));
#46463=CARTESIAN_POINT('',(195.5,-1.73686027918559,-14.0083302491977));
#46464=CARTESIAN_POINT('',(196.,-1.9206643666802,-14.4795611789942));
#46465=CARTESIAN_POINT('Origin',(190.,-1.60805974387778,-14.3674406716552));
#46466=CARTESIAN_POINT('',(190.,-1.47925920856997,-14.7265510941127));
#46467=CARTESIAN_POINT('',(190.,-1.73686027918559,-14.0083302491977));
#46468=CARTESIAN_POINT('',(190.,-3.22940520398334,-9.84694662451034));
#46469=CARTESIAN_POINT('',(190.,-1.73686027918559,-14.0083302491977));
#46470=CARTESIAN_POINT('',(190.,-1.47925920856997,-14.7265510941127));
#46471=CARTESIAN_POINT('Origin',(195.75,-4.2434301395928,-12.8498366001438));
#46472=CARTESIAN_POINT('',(196.,-4.3684301395928,-13.0663429510899));
#46473=CARTESIAN_POINT('',(195.5,-4.1184301395928,-12.6333302491977));
#46474=CARTESIAN_POINT('Origin',(190.,-18.6670488735913,-17.5127374981478));
#46475=CARTESIAN_POINT('',(190.5,-19.110417899636,-17.2646137433487));
#46476=CARTESIAN_POINT('',(190.5,-18.9951905283833,-17.900635094611));
#46477=CARTESIAN_POINT('',(190.5,-19.110417899636,-17.2646137433487));
#46478=CARTESIAN_POINT('',(190.,-18.6670488735913,-17.5127374981478));
#46479=CARTESIAN_POINT('',(190.,-18.6670488735913,-17.5127374981478));
#46480=CARTESIAN_POINT('',(190.5,-18.9951905283833,-17.900635094611));
#46481=CARTESIAN_POINT('Origin',(190.25,-13.3680367752315,-10.6825549777769));
#46482=CARTESIAN_POINT('',(190.,-13.1750260996004,-10.8414476430966));
#46483=CARTESIAN_POINT('',(190.5,-13.5610474508627,-10.5236623124571));
#46484=CARTESIAN_POINT('Origin',(195.5,-5.39638513844791,-25.182414249696));
#46485=CARTESIAN_POINT('',(195.5,-6.00480947161672,-25.400635094611));
#46486=CARTESIAN_POINT('',(196.,-5.83295112640873,-24.9225072872897));
#46487=CARTESIAN_POINT('',(195.5,-6.00480947161672,-25.400635094611));
#46488=CARTESIAN_POINT('',(195.5,-5.39638513844791,-25.182414249696));
#46489=CARTESIAN_POINT('',(195.5,-5.39638513844791,-25.182414249696));
#46490=CARTESIAN_POINT('',(196.,-5.83295112640874,-24.9225072872896));
#46491=CARTESIAN_POINT('Origin',(190.,-5.83295112640874,-24.9225072872897));
#46492=CARTESIAN_POINT('',(190.5,-6.00480947161672,-25.400635094611));
#46493=CARTESIAN_POINT('',(190.5,-5.39638513844791,-25.182414249696));
#46494=CARTESIAN_POINT('',(190.5,-6.00480947161672,-25.400635094611));
#46495=CARTESIAN_POINT('',(190.,-5.83295112640874,-24.9225072872897));
#46496=CARTESIAN_POINT('',(190.,-5.83295112640874,-24.9225072872897));
#46497=CARTESIAN_POINT('',(190.5,-5.39638513844791,-25.182414249696));
#46498=CARTESIAN_POINT('Origin',(190.25,-16.0556079660839,-19.3091287436648));
#46499=CARTESIAN_POINT('',(190.5,-16.1806079660839,-19.525635094611));
#46500=CARTESIAN_POINT('',(190.,-15.9306079660839,-19.0926223927187));
#46501=CARTESIAN_POINT('Origin',(190.25,-4.67248270213506,-22.5375143249309));
#46502=CARTESIAN_POINT('',(190.5,-4.43837227967758,-22.6252201405692));
#46503=CARTESIAN_POINT('',(190.,-4.90659312459254,-22.4498085092926));
#46504=CARTESIAN_POINT('Origin',(190.,-5.70059730503231,-25.2915246721535));
#46505=CARTESIAN_POINT('',(190.,-6.00480947161672,-25.400635094611));
#46506=CARTESIAN_POINT('',(190.,-5.39638513844791,-25.182414249696));
#46507=CARTESIAN_POINT('Origin',(195.75,-4.67248270213506,-22.5375143249309));
#46508=CARTESIAN_POINT('',(196.,-4.90659312459254,-22.4498085092926));
#46509=CARTESIAN_POINT('',(195.5,-4.43837227967758,-22.6252201405692));
#46510=CARTESIAN_POINT('Origin',(195.75,-16.0556079660839,-19.3091287436648));
#46511=CARTESIAN_POINT('',(196.,-15.9306079660839,-19.0926223927187));
#46512=CARTESIAN_POINT('',(195.5,-16.1806079660839,-19.525635094611));
#46513=CARTESIAN_POINT('Origin',(190.,-19.0528042140097,-17.5826244189798));
#46514=CARTESIAN_POINT('',(190.,-19.110417899636,-17.2646137433487));
#46515=CARTESIAN_POINT('',(190.,-18.9951905283833,-17.900635094611));
#46516=CARTESIAN_POINT('Origin',(195.75,-13.3680367752315,-10.6825549777769));
#46517=CARTESIAN_POINT('',(196.,-13.1750260996004,-10.8414476430966));
#46518=CARTESIAN_POINT('',(195.5,-13.5610474508627,-10.5236623124571));
#46519=CARTESIAN_POINT('Origin',(190.,-11.6961524227066,-8.25833024919769));
#46520=CARTESIAN_POINT('',(190.,-5.28794082615313,-0.47412417933778));
#46521=CARTESIAN_POINT('Origin',(190.,-1.30384757729338,-14.2583302491977));
#46522=CARTESIAN_POINT('',(190.,-0.151923788646696,-14.9233937586588));
#46523=CARTESIAN_POINT('Origin',(196.,-10.3660254037844,-16.9544826719043));
#46524=CARTESIAN_POINT('Origin',(190.,-19.4282032302755,-17.650635094611));
#46525=CARTESIAN_POINT('Ctrl Pts',(168.1,4.71844785465692E-15,25.));
#46526=CARTESIAN_POINT('Ctrl Pts',(168.1,0.490342890750044,25.));
#46527=CARTESIAN_POINT('Ctrl Pts',(168.197927739773,1.01300388320702,24.9841804475316));
#46528=CARTESIAN_POINT('Ctrl Pts',(168.595968837042,1.9730248402679,24.926626355682));
#46529=CARTESIAN_POINT('Ctrl Pts',(168.895370153156,2.41044277844561,24.886002008101));
#46530=CARTESIAN_POINT('Ctrl Pts',(169.587124183002,3.10037920374213,24.8094680053816));
#46531=CARTESIAN_POINT('Ctrl Pts',(170.463418858553,3.69742950735511,24.727449381457));
#46532=CARTESIAN_POINT('Ctrl Pts',(171.509209330769,3.8953602168609,24.694365273583));
#46533=CARTESIAN_POINT('Ctrl Pts',(172.429820467936,3.89494883801314,24.6944680938334));
#46534=CARTESIAN_POINT('Ctrl Pts',(173.337625674135,3.74893731769736,24.7187859134922));
#46535=CARTESIAN_POINT('Ctrl Pts',(174.346236594584,3.16619529082572,24.8015572991169));
#46536=CARTESIAN_POINT('Ctrl Pts',(174.958007340146,2.56739388230451,24.8693513631287));
#46537=CARTESIAN_POINT('Ctrl Pts',(175.489157477974,1.84426230866362,24.937097682422));
#46538=CARTESIAN_POINT('Ctrl Pts',(175.782240123002,1.08365275900373,24.9819016623594));
#46539=CARTESIAN_POINT('Ctrl Pts',(175.882356256358,0.418804816251774,24.9973027627956));
#46540=CARTESIAN_POINT('Ctrl Pts',(175.909743056997,-0.0151962230191145,
25.0015962526685));
#46541=CARTESIAN_POINT('Ctrl Pts',(175.870653276153,-0.779198836510287,
24.995496028175));
#46542=CARTESIAN_POINT('Ctrl Pts',(175.349399920632,-2.33707446060684,24.9151419492839));
#46543=CARTESIAN_POINT('Ctrl Pts',(174.336500109069,-3.24570229252571,24.790351880959));
#46544=CARTESIAN_POINT('Ctrl Pts',(173.254085442162,-3.6963447003694,24.7252038218524));
#46545=CARTESIAN_POINT('Ctrl Pts',(172.752744962911,-3.8461850836113,24.7021619625942));
#46546=CARTESIAN_POINT('Ctrl Pts',(172.245040749362,-3.89326696112091,24.6947095740839));
#46547=CARTESIAN_POINT('Ctrl Pts',(171.508328520708,-3.89399419357905,24.6944572637537));
#46548=CARTESIAN_POINT('Ctrl Pts',(170.985290745162,-3.79588962505944,24.7105170302552));
#46549=CARTESIAN_POINT('Ctrl Pts',(170.143631676592,-3.44706604659973,24.7613408689562));
#46550=CARTESIAN_POINT('Ctrl Pts',(169.472757569434,-3.03716583184694,24.8179083643489));
#46551=CARTESIAN_POINT('Ctrl Pts',(168.855166000548,-2.3552917259163,24.8917927252736));
#46552=CARTESIAN_POINT('Ctrl Pts',(168.267431880558,-1.33721306717284,24.9721836184323));
#46553=CARTESIAN_POINT('Ctrl Pts',(168.1,-0.55163791047639,25.));
#46554=CARTESIAN_POINT('Ctrl Pts',(168.1,-5.27355936696949E-15,25.));
#46555=CARTESIAN_POINT('Ctrl Pts',(168.266666666667,5.18104078158406E-15,
24.8333333333333));
#46556=CARTESIAN_POINT('Ctrl Pts',(168.266794313848,0.46646552227959,24.8332945640787));
#46557=CARTESIAN_POINT('Ctrl Pts',(168.359180904007,0.963922026904903,24.8188633380089));
#46558=CARTESIAN_POINT('Ctrl Pts',(168.736647912911,1.87993410901415,24.7661135751049));
#46559=CARTESIAN_POINT('Ctrl Pts',(169.021233517307,2.29895226345512,24.7288087600252));
#46560=CARTESIAN_POINT('Ctrl Pts',(169.681526448759,2.96173987210032,24.6583672833831));
#46561=CARTESIAN_POINT('Ctrl Pts',(170.520653439136,3.53818245366667,24.5826826921013));
#46562=CARTESIAN_POINT('Ctrl Pts',(171.527523707823,3.73046459774516,24.552046576372));
#46563=CARTESIAN_POINT('Ctrl Pts',(172.413771265711,3.73012216169543,24.5521081449956));
#46564=CARTESIAN_POINT('Ctrl Pts',(173.287906724152,3.5882347276893,24.5746675296835));
#46565=CARTESIAN_POINT('Ctrl Pts',(174.254886758977,3.02511186587481,24.6510708296085));
#46566=CARTESIAN_POINT('Ctrl Pts',(174.838876351617,2.44963017461608,24.7134857403187));
#46567=CARTESIAN_POINT('Ctrl Pts',(175.34440855413,1.7566933645737,24.7757283812278));
#46568=CARTESIAN_POINT('Ctrl Pts',(175.62192885337,1.03127566426168,24.8167727108676));
#46569=CARTESIAN_POINT('Ctrl Pts',(175.716614807647,0.398528431220379,24.8308669619708));
#46570=CARTESIAN_POINT('Ctrl Pts',(175.74268254159,-0.0144929189767075,
24.834825400553));
#46571=CARTESIAN_POINT('Ctrl Pts',(175.705398994411,-0.741374199846019,
24.8291900085961));
#46572=CARTESIAN_POINT('Ctrl Pts',(175.212629384802,-2.22576153108993,24.7557075376013));
#46573=CARTESIAN_POINT('Ctrl Pts',(174.246508948037,-3.10188851295124,24.6407628837638));
#46574=CARTESIAN_POINT('Ctrl Pts',(173.206751709011,-3.53753804437446,24.5805554974687));
#46575=CARTESIAN_POINT('Ctrl Pts',(172.724760251488,-3.68273779709261,24.5592626343764));
#46576=CARTESIAN_POINT('Ctrl Pts',(172.235889172339,-3.72837740200832,24.5523529001695));
#46577=CARTESIAN_POINT('Ctrl Pts',(171.526624153034,-3.72910914453677,24.5521281243884));
#46578=CARTESIAN_POINT('Ctrl Pts',(171.023033964314,-3.63384469616512,24.5669908902667));
#46579=CARTESIAN_POINT('Ctrl Pts',(170.21475055214,-3.29646898944012,24.6139400570373));
#46580=CARTESIAN_POINT('Ctrl Pts',(169.571724746233,-2.90061882815568,24.6661617079234));
#46581=CARTESIAN_POINT('Ctrl Pts',(168.983106184116,-2.24590741304073,24.7341018810264));
#46582=CARTESIAN_POINT('Ctrl Pts',(168.424797307501,-1.27242652685453,24.8078743314681));
#46583=CARTESIAN_POINT('Ctrl Pts',(168.266819442733,-0.524653038198594,
24.8332660143837));
#46584=CARTESIAN_POINT('Ctrl Pts',(168.266666666667,-4.92661467177413E-15,
24.8333333333333));
#46585=CARTESIAN_POINT('Ctrl Pts',(168.433333333333,5.64363370851121E-15,
24.6666666666667));
#46586=CARTESIAN_POINT('Ctrl Pts',(168.433205686152,0.442806217695906,24.6667054359213));
#46587=CARTESIAN_POINT('Ctrl Pts',(168.520379536409,0.91470391372393,24.6535646536479));
#46588=CARTESIAN_POINT('Ctrl Pts',(168.877269223955,1.78698013807251,24.6056117012029));
#46589=CARTESIAN_POINT('Ctrl Pts',(169.146992671644,2.1872659561253,24.5716344807208));
#46590=CARTESIAN_POINT('Ctrl Pts',(169.775922003246,2.82331390133092,24.5072699203476));
#46591=CARTESIAN_POINT('Ctrl Pts',(170.577934640553,3.37899466011285,24.4379056542893));
#46592=CARTESIAN_POINT('Ctrl Pts',(171.545724932034,3.56573461402839,24.4097113651223));
#46593=CARTESIAN_POINT('Ctrl Pts',(172.397850870814,3.56527124811576,24.4098336919766));
#46594=CARTESIAN_POINT('Ctrl Pts',(173.238134781157,3.42758948674762,24.4305206134708));
#46595=CARTESIAN_POINT('Ctrl Pts',(174.163594379135,2.88409824873316,24.5006229869098));
#46596=CARTESIAN_POINT('Ctrl Pts',(174.719788670977,2.33179149336597,24.5576379696713));
#46597=CARTESIAN_POINT('Ctrl Pts',(175.199753282856,1.66921727355042,24.6143923044647));
#46598=CARTESIAN_POINT('Ctrl Pts',(175.461540937543,0.978935543629066,24.6516390819393));
#46599=CARTESIAN_POINT('Ctrl Pts',(175.550908639782,0.378121403509141,24.6644241544695));
#46600=CARTESIAN_POINT('Ctrl Pts',(175.575182231976,-0.013759292292757,
24.6679615551863));
#46601=CARTESIAN_POINT('Ctrl Pts',(175.54045160512,-0.703288512377423,24.6629300098085));
#46602=CARTESIAN_POINT('Ctrl Pts',(175.075553895695,-2.11484158369124,24.5962216033143));
#46603=CARTESIAN_POINT('Ctrl Pts',(174.156435039991,-2.95775050705498,24.4912024202838));
#46604=CARTESIAN_POINT('Ctrl Pts',(173.159523604679,-3.37904065905067,24.435945095832));
#46605=CARTESIAN_POINT('Ctrl Pts',(172.696689494759,-3.51943249259346,24.4163697846433));
#46606=CARTESIAN_POINT('Ctrl Pts',(172.22679180891,-3.56372681457438,24.4100388485919));
#46607=CARTESIAN_POINT('Ctrl Pts',(171.544865156729,-3.56444742418653,24.4098140012409));
#46608=CARTESIAN_POINT('Ctrl Pts',(171.060891525884,-3.47208196124947,24.4234898517845));
#46609=CARTESIAN_POINT('Ctrl Pts',(170.285774210988,-3.14615677796927,24.4665898256047));
#46610=CARTESIAN_POINT('Ctrl Pts',(169.670874519592,-2.7645296126956,24.5144289115002));
#46611=CARTESIAN_POINT('Ctrl Pts',(169.110734773122,-2.13677771520377,24.5765207741377));
#46612=CARTESIAN_POINT('Ctrl Pts',(168.581809251079,-1.20782067924886,24.6436651038428));
#46613=CARTESIAN_POINT('Ctrl Pts',(168.433180557267,-0.498281671690027,
24.6667339856163));
#46614=CARTESIAN_POINT('Ctrl Pts',(168.433333333333,-4.57966997657877E-15,
24.6666666666667));
#46615=CARTESIAN_POINT('Ctrl Pts',(168.6,6.10622663543836E-15,24.5));
#46616=CARTESIAN_POINT('Ctrl Pts',(168.6,0.418928849225452,24.5));
#46617=CARTESIAN_POINT('Ctrl Pts',(168.681632700643,0.865622057421811,24.4882475441252));
#46618=CARTESIAN_POINT('Ctrl Pts',(169.017948299824,1.69388940681876,24.4450989206258));
#46619=CARTESIAN_POINT('Ctrl Pts',(169.272856035795,2.07577544113481,24.414441232645));
#46620=CARTESIAN_POINT('Ctrl Pts',(169.870324269003,2.68467456968911,24.3561691983492));
#46621=CARTESIAN_POINT('Ctrl Pts',(170.635169221136,3.21974760642441,24.2931389649336));
#46622=CARTESIAN_POINT('Ctrl Pts',(171.564039309088,3.40083899491265,24.2673926679114));
#46623=CARTESIAN_POINT('Ctrl Pts',(172.38180166859,3.40044457179805,24.2674737431389));
#46624=CARTESIAN_POINT('Ctrl Pts',(173.188415831174,3.26688689673955,24.286402229662));
#46625=CARTESIAN_POINT('Ctrl Pts',(174.072244543528,2.74301482378225,24.3501365174014));
#46626=CARTESIAN_POINT('Ctrl Pts',(174.600657682448,2.21402778567754,24.4017723468613));
#46627=CARTESIAN_POINT('Ctrl Pts',(175.055004359013,1.5816483294605,24.4530230032705));
#46628=CARTESIAN_POINT('Ctrl Pts',(175.301229667911,0.926558448887017,24.4865101304475));
#46629=CARTESIAN_POINT('Ctrl Pts',(175.385167191071,0.357845018477747,24.4979883536447));
#46630=CARTESIAN_POINT('Ctrl Pts',(175.408121716569,-0.01305598825035,24.5011907030708));
#46631=CARTESIAN_POINT('Ctrl Pts',(175.375197323378,-0.665463875713155,
24.4966239902296));
#46632=CARTESIAN_POINT('Ctrl Pts',(174.938783359865,-2.00352865417433,24.4367871916318));
#46633=CARTESIAN_POINT('Ctrl Pts',(174.066443878959,-2.81393672748051,24.3416134230885));
#46634=CARTESIAN_POINT('Ctrl Pts',(173.112189871528,-3.22023400305574,24.2912967714483));
#46635=CARTESIAN_POINT('Ctrl Pts',(172.668704783337,-3.35598520607476,24.2734704564255));
#46636=CARTESIAN_POINT('Ctrl Pts',(172.217640231887,-3.3988372554618,24.2676821746775));
#46637=CARTESIAN_POINT('Ctrl Pts',(171.563160789055,-3.39956237514424,24.2674848618756));
#46638=CARTESIAN_POINT('Ctrl Pts',(171.098634745036,-3.31003703235515,24.279963711796));
#46639=CARTESIAN_POINT('Ctrl Pts',(170.356893086536,-2.99555972080966,24.3191890136858));
#46640=CARTESIAN_POINT('Ctrl Pts',(169.769841696391,-2.62798260900435,24.3626822550747));
#46641=CARTESIAN_POINT('Ctrl Pts',(169.23867495669,-2.0273934023282,24.4188299298905));
#46642=CARTESIAN_POINT('Ctrl Pts',(168.739174678022,-1.14303413893055,24.4793558168787));
#46643=CARTESIAN_POINT('Ctrl Pts',(168.6,-0.471296799412231,24.5));
#46644=CARTESIAN_POINT('Ctrl Pts',(168.6,-4.23272528138341E-15,24.5));
#46645=CARTESIAN_POINT('',(168.6,6.10622663543836E-15,24.5));
#46646=CARTESIAN_POINT('',(168.1,4.71844785465692E-15,25.));
#46647=CARTESIAN_POINT('Ctrl Pts',(168.6,6.10622663543836E-15,24.5));
#46648=CARTESIAN_POINT('Ctrl Pts',(168.6,0.418928849225452,24.5));
#46649=CARTESIAN_POINT('Ctrl Pts',(168.681632700643,0.865622057421811,24.4882475441252));
#46650=CARTESIAN_POINT('Ctrl Pts',(169.017948299824,1.69388940681876,24.4450989206258));
#46651=CARTESIAN_POINT('Ctrl Pts',(169.272856035795,2.07577544113481,24.414441232645));
#46652=CARTESIAN_POINT('Ctrl Pts',(169.870324269003,2.68467456968911,24.3561691983492));
#46653=CARTESIAN_POINT('Ctrl Pts',(170.635169221136,3.21974760642441,24.2931389649336));
#46654=CARTESIAN_POINT('Ctrl Pts',(171.564039309088,3.40083899491265,24.2673926679114));
#46655=CARTESIAN_POINT('Ctrl Pts',(172.38180166859,3.40044457179805,24.2674737431389));
#46656=CARTESIAN_POINT('Ctrl Pts',(173.188415831174,3.26688689673955,24.286402229662));
#46657=CARTESIAN_POINT('Ctrl Pts',(174.072244543528,2.74301482378225,24.3501365174014));
#46658=CARTESIAN_POINT('Ctrl Pts',(174.600657682448,2.21402778567754,24.4017723468613));
#46659=CARTESIAN_POINT('Ctrl Pts',(175.055004359013,1.5816483294605,24.4530230032705));
#46660=CARTESIAN_POINT('Ctrl Pts',(175.301229667911,0.926558448887017,24.4865101304475));
#46661=CARTESIAN_POINT('Ctrl Pts',(175.385167191071,0.357845018477747,24.4979883536447));
#46662=CARTESIAN_POINT('Ctrl Pts',(175.408121716569,-0.01305598825035,24.5011907030708));
#46663=CARTESIAN_POINT('Ctrl Pts',(175.375197323378,-0.665463875713155,
24.4966239902296));
#46664=CARTESIAN_POINT('Ctrl Pts',(174.938783359865,-2.00352865417433,24.4367871916318));
#46665=CARTESIAN_POINT('Ctrl Pts',(174.066443878959,-2.81393672748051,24.3416134230885));
#46666=CARTESIAN_POINT('Ctrl Pts',(173.112189871528,-3.22023400305574,24.2912967714483));
#46667=CARTESIAN_POINT('Ctrl Pts',(172.668704783337,-3.35598520607476,24.2734704564255));
#46668=CARTESIAN_POINT('Ctrl Pts',(172.217640231887,-3.3988372554618,24.2676821746775));
#46669=CARTESIAN_POINT('Ctrl Pts',(171.563160789055,-3.39956237514424,24.2674848618756));
#46670=CARTESIAN_POINT('Ctrl Pts',(171.098634745036,-3.31003703235515,24.279963711796));
#46671=CARTESIAN_POINT('Ctrl Pts',(170.356893086536,-2.99555972080966,24.3191890136858));
#46672=CARTESIAN_POINT('Ctrl Pts',(169.769841696391,-2.62798260900435,24.3626822550747));
#46673=CARTESIAN_POINT('Ctrl Pts',(169.23867495669,-2.0273934023282,24.4188299298905));
#46674=CARTESIAN_POINT('Ctrl Pts',(168.739174678022,-1.14303413893055,24.4793558168787));
#46675=CARTESIAN_POINT('Ctrl Pts',(168.6,-0.471296799412231,24.5));
#46676=CARTESIAN_POINT('Ctrl Pts',(168.6,-4.23272528138341E-15,24.5));
#46677=CARTESIAN_POINT('Origin',(172.,0.,25.));
#46678=CARTESIAN_POINT('',(168.6,-4.163799117101E-16,10.));
#46679=CARTESIAN_POINT('',(168.6,4.163799117101E-16,25.));
#46680=CARTESIAN_POINT('',(175.4,0.,10.));
#46681=CARTESIAN_POINT('Origin',(172.,0.,10.));
#46682=CARTESIAN_POINT('Origin',(172.,0.,10.));
#46683=CARTESIAN_POINT('Origin',(172.,0.,10.));
#46684=CARTESIAN_POINT('',(175.,0.,10.));
#46685=CARTESIAN_POINT('Origin',(172.,0.,10.));
#46686=CARTESIAN_POINT('',(175.,0.,10.));
#46687=CARTESIAN_POINT('Origin',(190.,-5.5717967697245,-25.650635094611));
#46688=CARTESIAN_POINT('',(190.,-0.400087824116491,-11.8459522777201));
#46689=CARTESIAN_POINT('Origin',(190.,-10.3660254037844,-16.9544826719043));
#46690=CARTESIAN_POINT('Origin',(196.,-10.3660254037844,16.9544826719043));
#46691=CARTESIAN_POINT('Origin',(190.,25.,8.));
#46692=CARTESIAN_POINT('',(190.,17.0540540540541,6.67567567567568));
#46693=CARTESIAN_POINT('Origin',(190.,19.,0.));
#46694=CARTESIAN_POINT('Origin',(175.,0.,0.));
#46695=CARTESIAN_POINT('',(190.,6.12323399573677E-16,10.));
#46696=CARTESIAN_POINT('Origin',(190.,0.,0.));
#46697=CARTESIAN_POINT('',(175.,6.12323399573677E-16,10.));
#46698=CARTESIAN_POINT('',(175.,6.12323399573677E-16,10.));
#46699=CARTESIAN_POINT('Origin',(190.,10.,0.));
#55710=UNCERTAINTY_MEASURE_WITH_UNIT(LENGTH_MEASURE(0.01),#55738,
'DISTANCE_ACCURACY_VALUE',
'Maximum model space distance between geometric entities at asserted c
onnectivities');
#55715=UNCERTAINTY_MEASURE_WITH_UNIT(LENGTH_MEASURE(0.01),#55738,
'DISTANCE_ACCURACY_VALUE',
'Maximum model space distance between geometric entities at asserted c
onnectivities');
#55732=(
GEOMETRIC_REPRESENTATION_CONTEXT(3)
GLOBAL_UNCERTAINTY_ASSIGNED_CONTEXT((#55710))
GLOBAL_UNIT_ASSIGNED_CONTEXT((#55738,#55740,#55741))
REPRESENTATION_CONTEXT('','3D')
);
#55737=(
GEOMETRIC_REPRESENTATION_CONTEXT(3)
GLOBAL_UNCERTAINTY_ASSIGNED_CONTEXT((#55715))
GLOBAL_UNIT_ASSIGNED_CONTEXT((#55738,#55740,#55741))
REPRESENTATION_CONTEXT('','3D')
);
#55738=(
LENGTH_UNIT()
NAMED_UNIT(*)
SI_UNIT(.MILLI.,.METRE.)
);
#55740=(
NAMED_UNIT(*)
PLANE_ANGLE_UNIT()
SI_UNIT($,.RADIAN.)
);
#55741=(
NAMED_UNIT(*)
SI_UNIT($,.STERADIAN.)
SOLID_ANGLE_UNIT()
);
#55758=SHAPE_DEFINITION_REPRESENTATION(#55779,#55836);
#55779=PRODUCT_DEFINITION_SHAPE('',$,#55858);
#55836=SHAPE_REPRESENTATION('',(#29390),#55732);
#55841=PRODUCT_DEFINITION_CONTEXT('part definition',#55906,'design');
#55858=PRODUCT_DEFINITION('2026-10-26-00-34-41-330','20_Coupling_Hub',#55879,
#55841);
#55879=PRODUCT_DEFINITION_FORMATION('',$,#55924);
#55906=APPLICATION_CONTEXT(
'Core Data for Automotive Mechanical Design Process');
#55907=PRODUCT_CONTEXT('part definition',#55906,'mechanical');
#55924=PRODUCT('2026-10-26-00-34-41-330','20_Coupling_Hub',$,(#55907));
#55978=COLOUR_RGB('Sky Blue',0.24,0.69,0.87);
#55979=FILL_AREA_STYLE_COLOUR('',#55978);
#55980=FILL_AREA_STYLE('',(#55979));
#55981=SURFACE_STYLE_FILL_AREA(#55980);
#55982=SURFACE_SIDE_STYLE('',(#55981));
#55983=SURFACE_STYLE_USAGE(.BOTH.,#55982);
#55984=PRESENTATION_STYLE_ASSIGNMENT((#55983));
ENDSEC;
END-ISO-10303-21;
